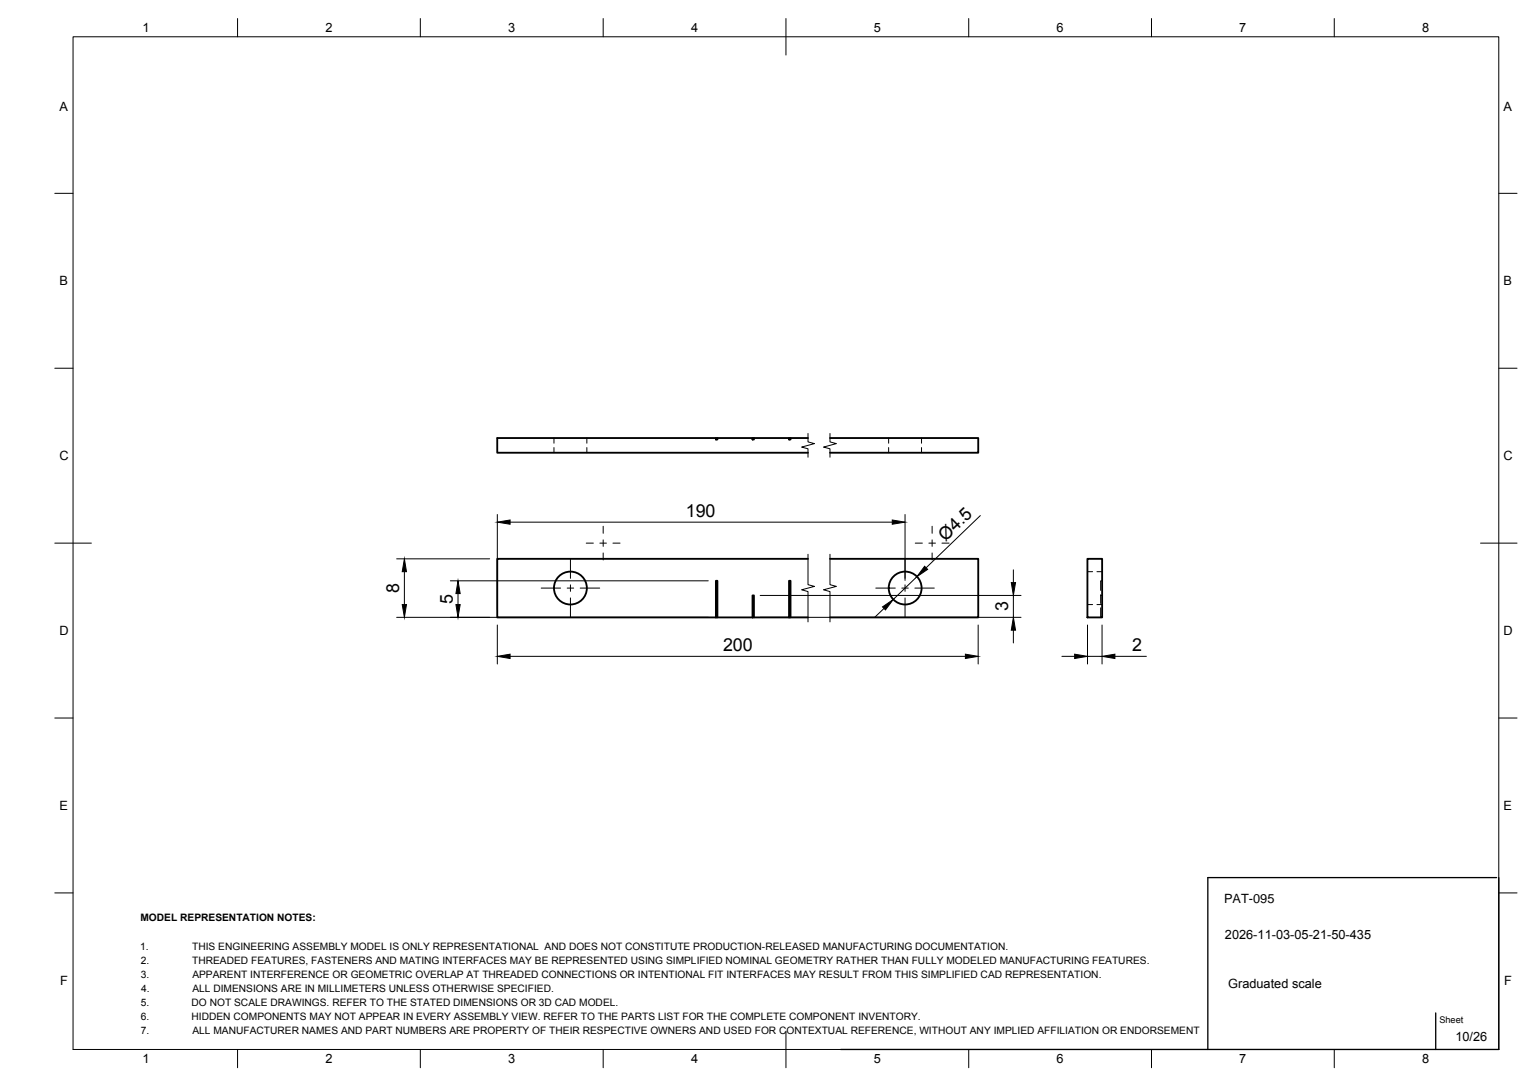
ISO-10303-21;
HEADER;
/* Generated by software containing ST-Developer
 * from STEP Tools, Inc. (www.steptools.com) 
 */

FILE_DESCRIPTION(
/* description */ ('Single-Axis Profile-Rail Linear Slide'),
/* implementation_level */ '2;1');

FILE_NAME(
/* name */ 'Graduated scale.step',
/* time_stamp */ '2026-10-27T10:47:43-07:00',
/* author */ (''),
/* organization */ (''),
/* preprocessor_version */ 'ST-DEVELOPER v20.2',
/* originating_system */ 'Autodesk Translation Framework v15.17.0.0',
/* authorisation */ '');

FILE_SCHEMA (('AUTOMOTIVE_DESIGN { 1 0 10303 214 3 1 1 }'));
ENDSEC;

DATA;
#10=MECHANICAL_DESIGN_GEOMETRIC_PRESENTATION_REPRESENTATION('',(#334),#14478);
#280=SHAPE_REPRESENTATION_RELATIONSHIP('SRR','None',#14610,#307);
#307=ADVANCED_BREP_SHAPE_REPRESENTATION('',(#361),#14454);
#334=STYLED_ITEM('',(#14845),#361);
#361=MANIFOLD_SOLID_BREP('Body1',#8594);
#418=FACE_BOUND('',#1508,.T.);
#419=FACE_BOUND('',#1509,.T.);
#420=FACE_BOUND('',#1517,.T.);
#421=FACE_BOUND('',#1518,.T.);
#502=PLANE('',#9027);
#503=PLANE('',#9028);
#504=PLANE('',#9029);
#505=PLANE('',#9030);
#506=PLANE('',#9031);
#507=PLANE('',#9032);
#508=PLANE('',#9033);
#509=PLANE('',#9034);
#510=PLANE('',#9035);
#511=PLANE('',#9036);
#512=PLANE('',#9037);
#513=PLANE('',#9038);
#514=PLANE('',#9039);
#515=PLANE('',#9040);
#516=PLANE('',#9041);
#517=PLANE('',#9042);
#518=PLANE('',#9043);
#519=PLANE('',#9044);
#520=PLANE('',#9045);
#521=PLANE('',#9046);
#522=PLANE('',#9047);
#523=PLANE('',#9048);
#524=PLANE('',#9049);
#525=PLANE('',#9050);
#526=PLANE('',#9051);
#527=PLANE('',#9052);
#528=PLANE('',#9053);
#529=PLANE('',#9054);
#530=PLANE('',#9055);
#531=PLANE('',#9056);
#532=PLANE('',#9057);
#533=PLANE('',#9058);
#534=PLANE('',#9059);
#535=PLANE('',#9060);
#536=PLANE('',#9061);
#537=PLANE('',#9062);
#538=PLANE('',#9063);
#539=PLANE('',#9064);
#540=PLANE('',#9065);
#541=PLANE('',#9066);
#542=PLANE('',#9067);
#543=PLANE('',#9068);
#544=PLANE('',#9069);
#545=PLANE('',#9070);
#546=PLANE('',#9071);
#547=PLANE('',#9072);
#548=PLANE('',#9073);
#549=PLANE('',#9074);
#550=PLANE('',#9075);
#551=PLANE('',#9076);
#552=PLANE('',#9077);
#553=PLANE('',#9078);
#554=PLANE('',#9079);
#555=PLANE('',#9080);
#556=PLANE('',#9081);
#557=PLANE('',#9082);
#558=PLANE('',#9083);
#559=PLANE('',#9084);
#560=PLANE('',#9085);
#561=PLANE('',#9086);
#562=PLANE('',#9087);
#563=PLANE('',#9088);
#564=PLANE('',#9089);
#565=PLANE('',#9090);
#566=PLANE('',#9091);
#567=PLANE('',#9092);
#568=PLANE('',#9093);
#569=PLANE('',#9094);
#570=PLANE('',#9095);
#571=PLANE('',#9096);
#572=PLANE('',#9097);
#573=PLANE('',#9098);
#574=PLANE('',#9099);
#575=PLANE('',#9100);
#576=PLANE('',#9101);
#577=PLANE('',#9102);
#578=PLANE('',#9103);
#579=PLANE('',#9104);
#580=PLANE('',#9105);
#581=PLANE('',#9106);
#582=PLANE('',#9107);
#583=PLANE('',#9108);
#584=PLANE('',#9109);
#585=PLANE('',#9110);
#586=PLANE('',#9111);
#587=PLANE('',#9112);
#588=PLANE('',#9113);
#589=PLANE('',#9114);
#590=PLANE('',#9115);
#591=PLANE('',#9116);
#592=PLANE('',#9117);
#593=PLANE('',#9118);
#594=PLANE('',#9119);
#595=PLANE('',#9120);
#596=PLANE('',#9121);
#597=PLANE('',#9122);
#598=PLANE('',#9123);
#599=PLANE('',#9124);
#600=PLANE('',#9125);
#601=PLANE('',#9126);
#602=PLANE('',#9127);
#603=PLANE('',#9128);
#604=PLANE('',#9129);
#605=PLANE('',#9130);
#606=PLANE('',#9131);
#607=PLANE('',#9132);
#608=PLANE('',#9133);
#609=PLANE('',#9134);
#610=PLANE('',#9135);
#611=PLANE('',#9136);
#612=PLANE('',#9137);
#613=PLANE('',#9138);
#614=PLANE('',#9139);
#615=PLANE('',#9140);
#616=PLANE('',#9141);
#617=PLANE('',#9142);
#618=PLANE('',#9143);
#619=PLANE('',#9150);
#620=PLANE('',#9151);
#621=PLANE('',#9152);
#622=PLANE('',#9153);
#623=PLANE('',#9154);
#896=FACE_OUTER_BOUND('',#1391,.T.);
#897=FACE_OUTER_BOUND('',#1392,.T.);
#898=FACE_OUTER_BOUND('',#1393,.T.);
#899=FACE_OUTER_BOUND('',#1394,.T.);
#900=FACE_OUTER_BOUND('',#1395,.T.);
#901=FACE_OUTER_BOUND('',#1396,.T.);
#902=FACE_OUTER_BOUND('',#1397,.T.);
#903=FACE_OUTER_BOUND('',#1398,.T.);
#904=FACE_OUTER_BOUND('',#1399,.T.);
#905=FACE_OUTER_BOUND('',#1400,.T.);
#906=FACE_OUTER_BOUND('',#1401,.T.);
#907=FACE_OUTER_BOUND('',#1402,.T.);
#908=FACE_OUTER_BOUND('',#1403,.T.);
#909=FACE_OUTER_BOUND('',#1404,.T.);
#910=FACE_OUTER_BOUND('',#1405,.T.);
#911=FACE_OUTER_BOUND('',#1406,.T.);
#912=FACE_OUTER_BOUND('',#1407,.T.);
#913=FACE_OUTER_BOUND('',#1408,.T.);
#914=FACE_OUTER_BOUND('',#1409,.T.);
#915=FACE_OUTER_BOUND('',#1410,.T.);
#916=FACE_OUTER_BOUND('',#1411,.T.);
#917=FACE_OUTER_BOUND('',#1412,.T.);
#918=FACE_OUTER_BOUND('',#1413,.T.);
#919=FACE_OUTER_BOUND('',#1414,.T.);
#920=FACE_OUTER_BOUND('',#1415,.T.);
#921=FACE_OUTER_BOUND('',#1416,.T.);
#922=FACE_OUTER_BOUND('',#1417,.T.);
#923=FACE_OUTER_BOUND('',#1418,.T.);
#924=FACE_OUTER_BOUND('',#1419,.T.);
#925=FACE_OUTER_BOUND('',#1420,.T.);
#926=FACE_OUTER_BOUND('',#1421,.T.);
#927=FACE_OUTER_BOUND('',#1422,.T.);
#928=FACE_OUTER_BOUND('',#1423,.T.);
#929=FACE_OUTER_BOUND('',#1424,.T.);
#930=FACE_OUTER_BOUND('',#1425,.T.);
#931=FACE_OUTER_BOUND('',#1426,.T.);
#932=FACE_OUTER_BOUND('',#1427,.T.);
#933=FACE_OUTER_BOUND('',#1428,.T.);
#934=FACE_OUTER_BOUND('',#1429,.T.);
#935=FACE_OUTER_BOUND('',#1430,.T.);
#936=FACE_OUTER_BOUND('',#1431,.T.);
#937=FACE_OUTER_BOUND('',#1432,.T.);
#938=FACE_OUTER_BOUND('',#1433,.T.);
#939=FACE_OUTER_BOUND('',#1434,.T.);
#940=FACE_OUTER_BOUND('',#1435,.T.);
#941=FACE_OUTER_BOUND('',#1436,.T.);
#942=FACE_OUTER_BOUND('',#1437,.T.);
#943=FACE_OUTER_BOUND('',#1438,.T.);
#944=FACE_OUTER_BOUND('',#1439,.T.);
#945=FACE_OUTER_BOUND('',#1440,.T.);
#946=FACE_OUTER_BOUND('',#1441,.T.);
#947=FACE_OUTER_BOUND('',#1442,.T.);
#948=FACE_OUTER_BOUND('',#1443,.T.);
#949=FACE_OUTER_BOUND('',#1444,.T.);
#950=FACE_OUTER_BOUND('',#1445,.T.);
#951=FACE_OUTER_BOUND('',#1446,.T.);
#952=FACE_OUTER_BOUND('',#1447,.T.);
#953=FACE_OUTER_BOUND('',#1448,.T.);
#954=FACE_OUTER_BOUND('',#1449,.T.);
#955=FACE_OUTER_BOUND('',#1450,.T.);
#956=FACE_OUTER_BOUND('',#1451,.T.);
#957=FACE_OUTER_BOUND('',#1452,.T.);
#958=FACE_OUTER_BOUND('',#1453,.T.);
#959=FACE_OUTER_BOUND('',#1454,.T.);
#960=FACE_OUTER_BOUND('',#1455,.T.);
#961=FACE_OUTER_BOUND('',#1456,.T.);
#962=FACE_OUTER_BOUND('',#1457,.T.);
#963=FACE_OUTER_BOUND('',#1458,.T.);
#964=FACE_OUTER_BOUND('',#1459,.T.);
#965=FACE_OUTER_BOUND('',#1460,.T.);
#966=FACE_OUTER_BOUND('',#1461,.T.);
#967=FACE_OUTER_BOUND('',#1462,.T.);
#968=FACE_OUTER_BOUND('',#1463,.T.);
#969=FACE_OUTER_BOUND('',#1464,.T.);
#970=FACE_OUTER_BOUND('',#1465,.T.);
#971=FACE_OUTER_BOUND('',#1466,.T.);
#972=FACE_OUTER_BOUND('',#1467,.T.);
#973=FACE_OUTER_BOUND('',#1468,.T.);
#974=FACE_OUTER_BOUND('',#1469,.T.);
#975=FACE_OUTER_BOUND('',#1470,.T.);
#976=FACE_OUTER_BOUND('',#1471,.T.);
#977=FACE_OUTER_BOUND('',#1472,.T.);
#978=FACE_OUTER_BOUND('',#1473,.T.);
#979=FACE_OUTER_BOUND('',#1474,.T.);
#980=FACE_OUTER_BOUND('',#1475,.T.);
#981=FACE_OUTER_BOUND('',#1476,.T.);
#982=FACE_OUTER_BOUND('',#1477,.T.);
#983=FACE_OUTER_BOUND('',#1478,.T.);
#984=FACE_OUTER_BOUND('',#1479,.T.);
#985=FACE_OUTER_BOUND('',#1480,.T.);
#986=FACE_OUTER_BOUND('',#1481,.T.);
#987=FACE_OUTER_BOUND('',#1482,.T.);
#988=FACE_OUTER_BOUND('',#1483,.T.);
#989=FACE_OUTER_BOUND('',#1484,.T.);
#990=FACE_OUTER_BOUND('',#1485,.T.);
#991=FACE_OUTER_BOUND('',#1486,.T.);
#992=FACE_OUTER_BOUND('',#1487,.T.);
#993=FACE_OUTER_BOUND('',#1488,.T.);
#994=FACE_OUTER_BOUND('',#1489,.T.);
#995=FACE_OUTER_BOUND('',#1490,.T.);
#996=FACE_OUTER_BOUND('',#1491,.T.);
#997=FACE_OUTER_BOUND('',#1492,.T.);
#998=FACE_OUTER_BOUND('',#1493,.T.);
#999=FACE_OUTER_BOUND('',#1494,.T.);
#1000=FACE_OUTER_BOUND('',#1495,.T.);
#1001=FACE_OUTER_BOUND('',#1496,.T.);
#1002=FACE_OUTER_BOUND('',#1497,.T.);
#1003=FACE_OUTER_BOUND('',#1498,.T.);
#1004=FACE_OUTER_BOUND('',#1499,.T.);
#1005=FACE_OUTER_BOUND('',#1500,.T.);
#1006=FACE_OUTER_BOUND('',#1501,.T.);
#1007=FACE_OUTER_BOUND('',#1502,.T.);
#1008=FACE_OUTER_BOUND('',#1503,.T.);
#1009=FACE_OUTER_BOUND('',#1504,.T.);
#1010=FACE_OUTER_BOUND('',#1505,.T.);
#1011=FACE_OUTER_BOUND('',#1506,.T.);
#1012=FACE_OUTER_BOUND('',#1507,.T.);
#1013=FACE_OUTER_BOUND('',#1510,.T.);
#1014=FACE_OUTER_BOUND('',#1511,.T.);
#1015=FACE_OUTER_BOUND('',#1512,.T.);
#1016=FACE_OUTER_BOUND('',#1513,.T.);
#1017=FACE_OUTER_BOUND('',#1514,.T.);
#1018=FACE_OUTER_BOUND('',#1515,.T.);
#1019=FACE_OUTER_BOUND('',#1516,.T.);
#1391=EDGE_LOOP('',(#6065,#6066,#6067,#6068));
#1392=EDGE_LOOP('',(#6069,#6070,#6071,#6072));
#1393=EDGE_LOOP('',(#6073,#6074,#6075,#6076));
#1394=EDGE_LOOP('',(#6077,#6078,#6079,#6080));
#1395=EDGE_LOOP('',(#6081,#6082,#6083,#6084));
#1396=EDGE_LOOP('',(#6085,#6086,#6087,#6088));
#1397=EDGE_LOOP('',(#6089,#6090,#6091,#6092));
#1398=EDGE_LOOP('',(#6093,#6094,#6095,#6096));
#1399=EDGE_LOOP('',(#6097,#6098,#6099,#6100));
#1400=EDGE_LOOP('',(#6101,#6102,#6103,#6104));
#1401=EDGE_LOOP('',(#6105,#6106,#6107,#6108));
#1402=EDGE_LOOP('',(#6109,#6110,#6111,#6112));
#1403=EDGE_LOOP('',(#6113,#6114,#6115,#6116));
#1404=EDGE_LOOP('',(#6117,#6118,#6119,#6120));
#1405=EDGE_LOOP('',(#6121,#6122,#6123,#6124));
#1406=EDGE_LOOP('',(#6125,#6126,#6127,#6128));
#1407=EDGE_LOOP('',(#6129,#6130,#6131,#6132));
#1408=EDGE_LOOP('',(#6133,#6134,#6135,#6136));
#1409=EDGE_LOOP('',(#6137,#6138,#6139,#6140));
#1410=EDGE_LOOP('',(#6141,#6142,#6143,#6144));
#1411=EDGE_LOOP('',(#6145,#6146,#6147,#6148));
#1412=EDGE_LOOP('',(#6149,#6150,#6151,#6152));
#1413=EDGE_LOOP('',(#6153,#6154,#6155,#6156));
#1414=EDGE_LOOP('',(#6157,#6158,#6159,#6160));
#1415=EDGE_LOOP('',(#6161,#6162,#6163,#6164));
#1416=EDGE_LOOP('',(#6165,#6166,#6167,#6168));
#1417=EDGE_LOOP('',(#6169,#6170,#6171,#6172));
#1418=EDGE_LOOP('',(#6173,#6174,#6175,#6176));
#1419=EDGE_LOOP('',(#6177,#6178,#6179,#6180));
#1420=EDGE_LOOP('',(#6181,#6182,#6183,#6184));
#1421=EDGE_LOOP('',(#6185,#6186,#6187,#6188));
#1422=EDGE_LOOP('',(#6189,#6190,#6191,#6192));
#1423=EDGE_LOOP('',(#6193,#6194,#6195,#6196));
#1424=EDGE_LOOP('',(#6197,#6198,#6199,#6200));
#1425=EDGE_LOOP('',(#6201,#6202,#6203,#6204));
#1426=EDGE_LOOP('',(#6205,#6206,#6207,#6208));
#1427=EDGE_LOOP('',(#6209,#6210,#6211,#6212));
#1428=EDGE_LOOP('',(#6213,#6214,#6215,#6216));
#1429=EDGE_LOOP('',(#6217,#6218,#6219,#6220));
#1430=EDGE_LOOP('',(#6221,#6222,#6223,#6224));
#1431=EDGE_LOOP('',(#6225,#6226,#6227,#6228));
#1432=EDGE_LOOP('',(#6229,#6230,#6231,#6232));
#1433=EDGE_LOOP('',(#6233,#6234,#6235,#6236));
#1434=EDGE_LOOP('',(#6237,#6238,#6239,#6240));
#1435=EDGE_LOOP('',(#6241,#6242,#6243,#6244));
#1436=EDGE_LOOP('',(#6245,#6246,#6247,#6248));
#1437=EDGE_LOOP('',(#6249,#6250,#6251,#6252));
#1438=EDGE_LOOP('',(#6253,#6254,#6255,#6256));
#1439=EDGE_LOOP('',(#6257,#6258,#6259,#6260));
#1440=EDGE_LOOP('',(#6261,#6262,#6263,#6264));
#1441=EDGE_LOOP('',(#6265,#6266,#6267,#6268));
#1442=EDGE_LOOP('',(#6269,#6270,#6271,#6272));
#1443=EDGE_LOOP('',(#6273,#6274,#6275,#6276));
#1444=EDGE_LOOP('',(#6277,#6278,#6279,#6280));
#1445=EDGE_LOOP('',(#6281,#6282,#6283,#6284));
#1446=EDGE_LOOP('',(#6285,#6286,#6287,#6288));
#1447=EDGE_LOOP('',(#6289,#6290,#6291,#6292));
#1448=EDGE_LOOP('',(#6293,#6294,#6295,#6296));
#1449=EDGE_LOOP('',(#6297,#6298,#6299,#6300));
#1450=EDGE_LOOP('',(#6301,#6302,#6303,#6304));
#1451=EDGE_LOOP('',(#6305,#6306,#6307,#6308));
#1452=EDGE_LOOP('',(#6309,#6310,#6311,#6312));
#1453=EDGE_LOOP('',(#6313,#6314,#6315,#6316));
#1454=EDGE_LOOP('',(#6317,#6318,#6319,#6320));
#1455=EDGE_LOOP('',(#6321,#6322,#6323,#6324));
#1456=EDGE_LOOP('',(#6325,#6326,#6327,#6328));
#1457=EDGE_LOOP('',(#6329,#6330,#6331,#6332));
#1458=EDGE_LOOP('',(#6333,#6334,#6335,#6336));
#1459=EDGE_LOOP('',(#6337,#6338,#6339,#6340));
#1460=EDGE_LOOP('',(#6341,#6342,#6343,#6344));
#1461=EDGE_LOOP('',(#6345,#6346,#6347,#6348));
#1462=EDGE_LOOP('',(#6349,#6350,#6351,#6352));
#1463=EDGE_LOOP('',(#6353,#6354,#6355,#6356));
#1464=EDGE_LOOP('',(#6357,#6358,#6359,#6360));
#1465=EDGE_LOOP('',(#6361,#6362,#6363,#6364));
#1466=EDGE_LOOP('',(#6365,#6366,#6367,#6368));
#1467=EDGE_LOOP('',(#6369,#6370,#6371,#6372));
#1468=EDGE_LOOP('',(#6373,#6374,#6375,#6376));
#1469=EDGE_LOOP('',(#6377,#6378,#6379,#6380));
#1470=EDGE_LOOP('',(#6381,#6382,#6383,#6384));
#1471=EDGE_LOOP('',(#6385,#6386,#6387,#6388));
#1472=EDGE_LOOP('',(#6389,#6390,#6391,#6392));
#1473=EDGE_LOOP('',(#6393,#6394,#6395,#6396));
#1474=EDGE_LOOP('',(#6397,#6398,#6399,#6400));
#1475=EDGE_LOOP('',(#6401,#6402,#6403,#6404));
#1476=EDGE_LOOP('',(#6405,#6406,#6407,#6408));
#1477=EDGE_LOOP('',(#6409,#6410,#6411,#6412));
#1478=EDGE_LOOP('',(#6413,#6414,#6415,#6416));
#1479=EDGE_LOOP('',(#6417,#6418,#6419,#6420));
#1480=EDGE_LOOP('',(#6421,#6422,#6423,#6424));
#1481=EDGE_LOOP('',(#6425,#6426,#6427,#6428));
#1482=EDGE_LOOP('',(#6429,#6430,#6431,#6432));
#1483=EDGE_LOOP('',(#6433,#6434,#6435,#6436));
#1484=EDGE_LOOP('',(#6437,#6438,#6439,#6440));
#1485=EDGE_LOOP('',(#6441,#6442,#6443,#6444));
#1486=EDGE_LOOP('',(#6445,#6446,#6447,#6448));
#1487=EDGE_LOOP('',(#6449,#6450,#6451,#6452));
#1488=EDGE_LOOP('',(#6453,#6454,#6455,#6456));
#1489=EDGE_LOOP('',(#6457,#6458,#6459,#6460));
#1490=EDGE_LOOP('',(#6461,#6462,#6463,#6464));
#1491=EDGE_LOOP('',(#6465,#6466,#6467,#6468));
#1492=EDGE_LOOP('',(#6469,#6470,#6471,#6472));
#1493=EDGE_LOOP('',(#6473,#6474,#6475,#6476));
#1494=EDGE_LOOP('',(#6477,#6478,#6479,#6480));
#1495=EDGE_LOOP('',(#6481,#6482,#6483,#6484));
#1496=EDGE_LOOP('',(#6485,#6486,#6487,#6488));
#1497=EDGE_LOOP('',(#6489,#6490,#6491,#6492));
#1498=EDGE_LOOP('',(#6493,#6494,#6495,#6496));
#1499=EDGE_LOOP('',(#6497,#6498,#6499,#6500));
#1500=EDGE_LOOP('',(#6501,#6502,#6503,#6504));
#1501=EDGE_LOOP('',(#6505,#6506,#6507,#6508));
#1502=EDGE_LOOP('',(#6509,#6510,#6511,#6512));
#1503=EDGE_LOOP('',(#6513,#6514,#6515,#6516));
#1504=EDGE_LOOP('',(#6517,#6518,#6519,#6520));
#1505=EDGE_LOOP('',(#6521,#6522,#6523,#6524));
#1506=EDGE_LOOP('',(#6525,#6526,#6527,#6528));
#1507=EDGE_LOOP('',(#6529,#6530,#6531,#6532,#6533,#6534,#6535,#6536,#6537,
#6538,#6539,#6540,#6541,#6542,#6543,#6544,#6545,#6546,#6547,#6548,#6549,
#6550,#6551,#6552,#6553,#6554,#6555,#6556,#6557,#6558,#6559,#6560,#6561,
#6562,#6563,#6564,#6565,#6566,#6567,#6568,#6569,#6570,#6571,#6572,#6573,
#6574,#6575,#6576,#6577,#6578,#6579,#6580,#6581,#6582,#6583,#6584,#6585,
#6586,#6587,#6588,#6589,#6590,#6591,#6592,#6593,#6594,#6595,#6596,#6597,
#6598,#6599,#6600,#6601,#6602,#6603,#6604,#6605,#6606,#6607,#6608,#6609,
#6610,#6611,#6612,#6613,#6614,#6615,#6616,#6617,#6618,#6619,#6620,#6621,
#6622,#6623,#6624,#6625,#6626,#6627,#6628,#6629,#6630,#6631,#6632,#6633,
#6634,#6635,#6636,#6637,#6638,#6639,#6640,#6641,#6642,#6643,#6644,#6645,
#6646,#6647,#6648));
#1508=EDGE_LOOP('',(#6649));
#1509=EDGE_LOOP('',(#6650));
#1510=EDGE_LOOP('',(#6651,#6652,#6653,#6654));
#1511=EDGE_LOOP('',(#6655,#6656,#6657,#6658));
#1512=EDGE_LOOP('',(#6659,#6660,#6661,#6662));
#1513=EDGE_LOOP('',(#6663,#6664,#6665,#6666));
#1514=EDGE_LOOP('',(#6667,#6668,#6669,#6670,#6671,#6672,#6673,#6674,#6675,
#6676,#6677,#6678,#6679,#6680,#6681,#6682,#6683,#6684,#6685,#6686,#6687,
#6688,#6689,#6690,#6691,#6692,#6693,#6694,#6695,#6696,#6697,#6698,#6699,
#6700,#6701,#6702,#6703,#6704,#6705,#6706,#6707,#6708,#6709,#6710,#6711,
#6712,#6713,#6714,#6715,#6716,#6717,#6718,#6719,#6720,#6721,#6722,#6723,
#6724,#6725,#6726,#6727,#6728,#6729,#6730,#6731,#6732,#6733,#6734,#6735,
#6736,#6737,#6738,#6739,#6740,#6741,#6742,#6743,#6744,#6745,#6746,#6747,
#6748,#6749,#6750,#6751,#6752,#6753,#6754,#6755,#6756,#6757,#6758,#6759,
#6760,#6761,#6762,#6763,#6764,#6765,#6766,#6767,#6768,#6769,#6770,#6771,
#6772,#6773,#6774,#6775,#6776,#6777,#6778,#6779,#6780,#6781,#6782,#6783,
#6784,#6785,#6786));
#1515=EDGE_LOOP('',(#6787,#6788,#6789,#6790));
#1516=EDGE_LOOP('',(#6791,#6792,#6793,#6794));
#1517=EDGE_LOOP('',(#6795));
#1518=EDGE_LOOP('',(#6796));
#1922=LINE('',#12273,#2893);
#1923=LINE('',#12275,#2894);
#1924=LINE('',#12277,#2895);
#1925=LINE('',#12278,#2896);
#1926=LINE('',#12281,#2897);
#1927=LINE('',#12283,#2898);
#1928=LINE('',#12284,#2899);
#1929=LINE('',#12287,#2900);
#1930=LINE('',#12289,#2901);
#1931=LINE('',#12290,#2902);
#1932=LINE('',#12292,#2903);
#1933=LINE('',#12296,#2904);
#1934=LINE('',#12298,#2905);
#1935=LINE('',#12300,#2906);
#1936=LINE('',#12301,#2907);
#1937=LINE('',#12304,#2908);
#1938=LINE('',#12306,#2909);
#1939=LINE('',#12307,#2910);
#1940=LINE('',#12310,#2911);
#1941=LINE('',#12312,#2912);
#1942=LINE('',#12313,#2913);
#1943=LINE('',#12315,#2914);
#1944=LINE('',#12319,#2915);
#1945=LINE('',#12321,#2916);
#1946=LINE('',#12323,#2917);
#1947=LINE('',#12324,#2918);
#1948=LINE('',#12327,#2919);
#1949=LINE('',#12329,#2920);
#1950=LINE('',#12330,#2921);
#1951=LINE('',#12333,#2922);
#1952=LINE('',#12335,#2923);
#1953=LINE('',#12336,#2924);
#1954=LINE('',#12338,#2925);
#1955=LINE('',#12342,#2926);
#1956=LINE('',#12344,#2927);
#1957=LINE('',#12346,#2928);
#1958=LINE('',#12347,#2929);
#1959=LINE('',#12350,#2930);
#1960=LINE('',#12352,#2931);
#1961=LINE('',#12353,#2932);
#1962=LINE('',#12356,#2933);
#1963=LINE('',#12358,#2934);
#1964=LINE('',#12359,#2935);
#1965=LINE('',#12361,#2936);
#1966=LINE('',#12365,#2937);
#1967=LINE('',#12367,#2938);
#1968=LINE('',#12369,#2939);
#1969=LINE('',#12370,#2940);
#1970=LINE('',#12373,#2941);
#1971=LINE('',#12375,#2942);
#1972=LINE('',#12376,#2943);
#1973=LINE('',#12379,#2944);
#1974=LINE('',#12381,#2945);
#1975=LINE('',#12382,#2946);
#1976=LINE('',#12384,#2947);
#1977=LINE('',#12388,#2948);
#1978=LINE('',#12390,#2949);
#1979=LINE('',#12392,#2950);
#1980=LINE('',#12393,#2951);
#1981=LINE('',#12396,#2952);
#1982=LINE('',#12398,#2953);
#1983=LINE('',#12399,#2954);
#1984=LINE('',#12402,#2955);
#1985=LINE('',#12404,#2956);
#1986=LINE('',#12405,#2957);
#1987=LINE('',#12407,#2958);
#1988=LINE('',#12411,#2959);
#1989=LINE('',#12413,#2960);
#1990=LINE('',#12415,#2961);
#1991=LINE('',#12416,#2962);
#1992=LINE('',#12419,#2963);
#1993=LINE('',#12421,#2964);
#1994=LINE('',#12422,#2965);
#1995=LINE('',#12425,#2966);
#1996=LINE('',#12427,#2967);
#1997=LINE('',#12428,#2968);
#1998=LINE('',#12430,#2969);
#1999=LINE('',#12434,#2970);
#2000=LINE('',#12436,#2971);
#2001=LINE('',#12438,#2972);
#2002=LINE('',#12439,#2973);
#2003=LINE('',#12442,#2974);
#2004=LINE('',#12444,#2975);
#2005=LINE('',#12445,#2976);
#2006=LINE('',#12448,#2977);
#2007=LINE('',#12450,#2978);
#2008=LINE('',#12451,#2979);
#2009=LINE('',#12453,#2980);
#2010=LINE('',#12457,#2981);
#2011=LINE('',#12459,#2982);
#2012=LINE('',#12461,#2983);
#2013=LINE('',#12462,#2984);
#2014=LINE('',#12465,#2985);
#2015=LINE('',#12467,#2986);
#2016=LINE('',#12468,#2987);
#2017=LINE('',#12471,#2988);
#2018=LINE('',#12473,#2989);
#2019=LINE('',#12474,#2990);
#2020=LINE('',#12476,#2991);
#2021=LINE('',#12480,#2992);
#2022=LINE('',#12482,#2993);
#2023=LINE('',#12484,#2994);
#2024=LINE('',#12485,#2995);
#2025=LINE('',#12488,#2996);
#2026=LINE('',#12490,#2997);
#2027=LINE('',#12491,#2998);
#2028=LINE('',#12494,#2999);
#2029=LINE('',#12496,#3000);
#2030=LINE('',#12497,#3001);
#2031=LINE('',#12499,#3002);
#2032=LINE('',#12503,#3003);
#2033=LINE('',#12505,#3004);
#2034=LINE('',#12507,#3005);
#2035=LINE('',#12508,#3006);
#2036=LINE('',#12511,#3007);
#2037=LINE('',#12513,#3008);
#2038=LINE('',#12514,#3009);
#2039=LINE('',#12517,#3010);
#2040=LINE('',#12519,#3011);
#2041=LINE('',#12520,#3012);
#2042=LINE('',#12522,#3013);
#2043=LINE('',#12526,#3014);
#2044=LINE('',#12528,#3015);
#2045=LINE('',#12530,#3016);
#2046=LINE('',#12531,#3017);
#2047=LINE('',#12534,#3018);
#2048=LINE('',#12536,#3019);
#2049=LINE('',#12537,#3020);
#2050=LINE('',#12540,#3021);
#2051=LINE('',#12542,#3022);
#2052=LINE('',#12543,#3023);
#2053=LINE('',#12545,#3024);
#2054=LINE('',#12549,#3025);
#2055=LINE('',#12551,#3026);
#2056=LINE('',#12553,#3027);
#2057=LINE('',#12554,#3028);
#2058=LINE('',#12557,#3029);
#2059=LINE('',#12559,#3030);
#2060=LINE('',#12560,#3031);
#2061=LINE('',#12563,#3032);
#2062=LINE('',#12565,#3033);
#2063=LINE('',#12566,#3034);
#2064=LINE('',#12568,#3035);
#2065=LINE('',#12572,#3036);
#2066=LINE('',#12574,#3037);
#2067=LINE('',#12576,#3038);
#2068=LINE('',#12577,#3039);
#2069=LINE('',#12580,#3040);
#2070=LINE('',#12582,#3041);
#2071=LINE('',#12583,#3042);
#2072=LINE('',#12586,#3043);
#2073=LINE('',#12588,#3044);
#2074=LINE('',#12589,#3045);
#2075=LINE('',#12591,#3046);
#2076=LINE('',#12595,#3047);
#2077=LINE('',#12597,#3048);
#2078=LINE('',#12599,#3049);
#2079=LINE('',#12600,#3050);
#2080=LINE('',#12603,#3051);
#2081=LINE('',#12605,#3052);
#2082=LINE('',#12606,#3053);
#2083=LINE('',#12609,#3054);
#2084=LINE('',#12611,#3055);
#2085=LINE('',#12612,#3056);
#2086=LINE('',#12614,#3057);
#2087=LINE('',#12618,#3058);
#2088=LINE('',#12620,#3059);
#2089=LINE('',#12622,#3060);
#2090=LINE('',#12623,#3061);
#2091=LINE('',#12626,#3062);
#2092=LINE('',#12628,#3063);
#2093=LINE('',#12629,#3064);
#2094=LINE('',#12632,#3065);
#2095=LINE('',#12634,#3066);
#2096=LINE('',#12635,#3067);
#2097=LINE('',#12637,#3068);
#2098=LINE('',#12641,#3069);
#2099=LINE('',#12643,#3070);
#2100=LINE('',#12645,#3071);
#2101=LINE('',#12646,#3072);
#2102=LINE('',#12649,#3073);
#2103=LINE('',#12651,#3074);
#2104=LINE('',#12652,#3075);
#2105=LINE('',#12655,#3076);
#2106=LINE('',#12657,#3077);
#2107=LINE('',#12658,#3078);
#2108=LINE('',#12660,#3079);
#2109=LINE('',#12664,#3080);
#2110=LINE('',#12666,#3081);
#2111=LINE('',#12668,#3082);
#2112=LINE('',#12669,#3083);
#2113=LINE('',#12672,#3084);
#2114=LINE('',#12674,#3085);
#2115=LINE('',#12675,#3086);
#2116=LINE('',#12678,#3087);
#2117=LINE('',#12680,#3088);
#2118=LINE('',#12681,#3089);
#2119=LINE('',#12683,#3090);
#2120=LINE('',#12687,#3091);
#2121=LINE('',#12689,#3092);
#2122=LINE('',#12691,#3093);
#2123=LINE('',#12692,#3094);
#2124=LINE('',#12695,#3095);
#2125=LINE('',#12697,#3096);
#2126=LINE('',#12698,#3097);
#2127=LINE('',#12701,#3098);
#2128=LINE('',#12703,#3099);
#2129=LINE('',#12704,#3100);
#2130=LINE('',#12706,#3101);
#2131=LINE('',#12710,#3102);
#2132=LINE('',#12712,#3103);
#2133=LINE('',#12714,#3104);
#2134=LINE('',#12715,#3105);
#2135=LINE('',#12718,#3106);
#2136=LINE('',#12720,#3107);
#2137=LINE('',#12721,#3108);
#2138=LINE('',#12724,#3109);
#2139=LINE('',#12726,#3110);
#2140=LINE('',#12727,#3111);
#2141=LINE('',#12729,#3112);
#2142=LINE('',#12733,#3113);
#2143=LINE('',#12735,#3114);
#2144=LINE('',#12737,#3115);
#2145=LINE('',#12738,#3116);
#2146=LINE('',#12741,#3117);
#2147=LINE('',#12743,#3118);
#2148=LINE('',#12744,#3119);
#2149=LINE('',#12747,#3120);
#2150=LINE('',#12749,#3121);
#2151=LINE('',#12750,#3122);
#2152=LINE('',#12752,#3123);
#2153=LINE('',#12756,#3124);
#2154=LINE('',#12758,#3125);
#2155=LINE('',#12760,#3126);
#2156=LINE('',#12761,#3127);
#2157=LINE('',#12764,#3128);
#2158=LINE('',#12766,#3129);
#2159=LINE('',#12767,#3130);
#2160=LINE('',#12770,#3131);
#2161=LINE('',#12772,#3132);
#2162=LINE('',#12773,#3133);
#2163=LINE('',#12775,#3134);
#2164=LINE('',#12779,#3135);
#2165=LINE('',#12781,#3136);
#2166=LINE('',#12783,#3137);
#2167=LINE('',#12784,#3138);
#2168=LINE('',#12787,#3139);
#2169=LINE('',#12789,#3140);
#2170=LINE('',#12790,#3141);
#2171=LINE('',#12793,#3142);
#2172=LINE('',#12795,#3143);
#2173=LINE('',#12796,#3144);
#2174=LINE('',#12798,#3145);
#2175=LINE('',#12802,#3146);
#2176=LINE('',#12804,#3147);
#2177=LINE('',#12806,#3148);
#2178=LINE('',#12807,#3149);
#2179=LINE('',#12810,#3150);
#2180=LINE('',#12812,#3151);
#2181=LINE('',#12813,#3152);
#2182=LINE('',#12816,#3153);
#2183=LINE('',#12818,#3154);
#2184=LINE('',#12819,#3155);
#2185=LINE('',#12821,#3156);
#2186=LINE('',#12825,#3157);
#2187=LINE('',#12827,#3158);
#2188=LINE('',#12829,#3159);
#2189=LINE('',#12830,#3160);
#2190=LINE('',#12833,#3161);
#2191=LINE('',#12835,#3162);
#2192=LINE('',#12836,#3163);
#2193=LINE('',#12839,#3164);
#2194=LINE('',#12841,#3165);
#2195=LINE('',#12842,#3166);
#2196=LINE('',#12844,#3167);
#2197=LINE('',#12848,#3168);
#2198=LINE('',#12850,#3169);
#2199=LINE('',#12852,#3170);
#2200=LINE('',#12853,#3171);
#2201=LINE('',#12856,#3172);
#2202=LINE('',#12858,#3173);
#2203=LINE('',#12859,#3174);
#2204=LINE('',#12862,#3175);
#2205=LINE('',#12864,#3176);
#2206=LINE('',#12865,#3177);
#2207=LINE('',#12867,#3178);
#2208=LINE('',#12871,#3179);
#2209=LINE('',#12873,#3180);
#2210=LINE('',#12875,#3181);
#2211=LINE('',#12876,#3182);
#2212=LINE('',#12879,#3183);
#2213=LINE('',#12881,#3184);
#2214=LINE('',#12882,#3185);
#2215=LINE('',#12885,#3186);
#2216=LINE('',#12887,#3187);
#2217=LINE('',#12888,#3188);
#2218=LINE('',#12890,#3189);
#2219=LINE('',#12894,#3190);
#2220=LINE('',#12896,#3191);
#2221=LINE('',#12898,#3192);
#2222=LINE('',#12899,#3193);
#2223=LINE('',#12902,#3194);
#2224=LINE('',#12904,#3195);
#2225=LINE('',#12905,#3196);
#2226=LINE('',#12908,#3197);
#2227=LINE('',#12910,#3198);
#2228=LINE('',#12911,#3199);
#2229=LINE('',#12913,#3200);
#2230=LINE('',#12917,#3201);
#2231=LINE('',#12919,#3202);
#2232=LINE('',#12921,#3203);
#2233=LINE('',#12922,#3204);
#2234=LINE('',#12925,#3205);
#2235=LINE('',#12927,#3206);
#2236=LINE('',#12928,#3207);
#2237=LINE('',#12931,#3208);
#2238=LINE('',#12933,#3209);
#2239=LINE('',#12934,#3210);
#2240=LINE('',#12936,#3211);
#2241=LINE('',#12938,#3212);
#2242=LINE('',#12940,#3213);
#2243=LINE('',#12942,#3214);
#2244=LINE('',#12944,#3215);
#2245=LINE('',#12946,#3216);
#2246=LINE('',#12947,#3217);
#2247=LINE('',#12948,#3218);
#2248=LINE('',#12949,#3219);
#2249=LINE('',#12950,#3220);
#2250=LINE('',#12951,#3221);
#2251=LINE('',#12952,#3222);
#2252=LINE('',#12953,#3223);
#2253=LINE('',#12954,#3224);
#2254=LINE('',#12955,#3225);
#2255=LINE('',#12956,#3226);
#2256=LINE('',#12957,#3227);
#2257=LINE('',#12958,#3228);
#2258=LINE('',#12959,#3229);
#2259=LINE('',#12960,#3230);
#2260=LINE('',#12961,#3231);
#2261=LINE('',#12962,#3232);
#2262=LINE('',#12963,#3233);
#2263=LINE('',#12964,#3234);
#2264=LINE('',#12965,#3235);
#2265=LINE('',#12966,#3236);
#2266=LINE('',#12967,#3237);
#2267=LINE('',#12968,#3238);
#2268=LINE('',#12969,#3239);
#2269=LINE('',#12970,#3240);
#2270=LINE('',#12971,#3241);
#2271=LINE('',#12972,#3242);
#2272=LINE('',#12973,#3243);
#2273=LINE('',#12974,#3244);
#2274=LINE('',#12982,#3245);
#2275=LINE('',#12986,#3246);
#2276=LINE('',#12990,#3247);
#2277=LINE('',#12991,#3248);
#2278=LINE('',#12992,#3249);
#2279=LINE('',#12995,#3250);
#2280=LINE('',#12996,#3251);
#2281=LINE('',#12999,#3252);
#2282=LINE('',#13000,#3253);
#2283=LINE('',#13002,#3254);
#2893=VECTOR('',#9921,1.);
#2894=VECTOR('',#9922,1.);
#2895=VECTOR('',#9923,1.);
#2896=VECTOR('',#9924,1.);
#2897=VECTOR('',#9927,1.);
#2898=VECTOR('',#9928,1.);
#2899=VECTOR('',#9929,1.);
#2900=VECTOR('',#9932,1.);
#2901=VECTOR('',#9933,1.);
#2902=VECTOR('',#9934,1.);
#2903=VECTOR('',#9937,1.);
#2904=VECTOR('',#9940,1.);
#2905=VECTOR('',#9941,1.);
#2906=VECTOR('',#9942,1.);
#2907=VECTOR('',#9943,1.);
#2908=VECTOR('',#9946,1.);
#2909=VECTOR('',#9947,1.);
#2910=VECTOR('',#9948,1.);
#2911=VECTOR('',#9951,1.);
#2912=VECTOR('',#9952,1.);
#2913=VECTOR('',#9953,1.);
#2914=VECTOR('',#9956,1.);
#2915=VECTOR('',#9959,1.);
#2916=VECTOR('',#9960,1.);
#2917=VECTOR('',#9961,1.);
#2918=VECTOR('',#9962,1.);
#2919=VECTOR('',#9965,1.);
#2920=VECTOR('',#9966,1.);
#2921=VECTOR('',#9967,1.);
#2922=VECTOR('',#9970,1.);
#2923=VECTOR('',#9971,1.);
#2924=VECTOR('',#9972,1.);
#2925=VECTOR('',#9975,1.);
#2926=VECTOR('',#9978,1.);
#2927=VECTOR('',#9979,1.);
#2928=VECTOR('',#9980,1.);
#2929=VECTOR('',#9981,1.);
#2930=VECTOR('',#9984,1.);
#2931=VECTOR('',#9985,1.);
#2932=VECTOR('',#9986,1.);
#2933=VECTOR('',#9989,1.);
#2934=VECTOR('',#9990,1.);
#2935=VECTOR('',#9991,1.);
#2936=VECTOR('',#9994,1.);
#2937=VECTOR('',#9997,1.);
#2938=VECTOR('',#9998,1.);
#2939=VECTOR('',#9999,1.);
#2940=VECTOR('',#10000,1.);
#2941=VECTOR('',#10003,1.);
#2942=VECTOR('',#10004,1.);
#2943=VECTOR('',#10005,1.);
#2944=VECTOR('',#10008,1.);
#2945=VECTOR('',#10009,1.);
#2946=VECTOR('',#10010,1.);
#2947=VECTOR('',#10013,1.);
#2948=VECTOR('',#10016,1.);
#2949=VECTOR('',#10017,1.);
#2950=VECTOR('',#10018,1.);
#2951=VECTOR('',#10019,1.);
#2952=VECTOR('',#10022,1.);
#2953=VECTOR('',#10023,1.);
#2954=VECTOR('',#10024,1.);
#2955=VECTOR('',#10027,1.);
#2956=VECTOR('',#10028,1.);
#2957=VECTOR('',#10029,1.);
#2958=VECTOR('',#10032,1.);
#2959=VECTOR('',#10035,1.);
#2960=VECTOR('',#10036,1.);
#2961=VECTOR('',#10037,1.);
#2962=VECTOR('',#10038,1.);
#2963=VECTOR('',#10041,1.);
#2964=VECTOR('',#10042,1.);
#2965=VECTOR('',#10043,1.);
#2966=VECTOR('',#10046,1.);
#2967=VECTOR('',#10047,1.);
#2968=VECTOR('',#10048,1.);
#2969=VECTOR('',#10051,1.);
#2970=VECTOR('',#10054,1.);
#2971=VECTOR('',#10055,1.);
#2972=VECTOR('',#10056,1.);
#2973=VECTOR('',#10057,1.);
#2974=VECTOR('',#10060,1.);
#2975=VECTOR('',#10061,1.);
#2976=VECTOR('',#10062,1.);
#2977=VECTOR('',#10065,1.);
#2978=VECTOR('',#10066,1.);
#2979=VECTOR('',#10067,1.);
#2980=VECTOR('',#10070,1.);
#2981=VECTOR('',#10073,1.);
#2982=VECTOR('',#10074,1.);
#2983=VECTOR('',#10075,1.);
#2984=VECTOR('',#10076,1.);
#2985=VECTOR('',#10079,1.);
#2986=VECTOR('',#10080,1.);
#2987=VECTOR('',#10081,1.);
#2988=VECTOR('',#10084,1.);
#2989=VECTOR('',#10085,1.);
#2990=VECTOR('',#10086,1.);
#2991=VECTOR('',#10089,1.);
#2992=VECTOR('',#10092,1.);
#2993=VECTOR('',#10093,1.);
#2994=VECTOR('',#10094,1.);
#2995=VECTOR('',#10095,1.);
#2996=VECTOR('',#10098,1.);
#2997=VECTOR('',#10099,1.);
#2998=VECTOR('',#10100,1.);
#2999=VECTOR('',#10103,1.);
#3000=VECTOR('',#10104,1.);
#3001=VECTOR('',#10105,1.);
#3002=VECTOR('',#10108,1.);
#3003=VECTOR('',#10111,1.);
#3004=VECTOR('',#10112,1.);
#3005=VECTOR('',#10113,1.);
#3006=VECTOR('',#10114,1.);
#3007=VECTOR('',#10117,1.);
#3008=VECTOR('',#10118,1.);
#3009=VECTOR('',#10119,1.);
#3010=VECTOR('',#10122,1.);
#3011=VECTOR('',#10123,1.);
#3012=VECTOR('',#10124,1.);
#3013=VECTOR('',#10127,1.);
#3014=VECTOR('',#10130,1.);
#3015=VECTOR('',#10131,1.);
#3016=VECTOR('',#10132,1.);
#3017=VECTOR('',#10133,1.);
#3018=VECTOR('',#10136,1.);
#3019=VECTOR('',#10137,1.);
#3020=VECTOR('',#10138,1.);
#3021=VECTOR('',#10141,1.);
#3022=VECTOR('',#10142,1.);
#3023=VECTOR('',#10143,1.);
#3024=VECTOR('',#10146,1.);
#3025=VECTOR('',#10149,1.);
#3026=VECTOR('',#10150,1.);
#3027=VECTOR('',#10151,1.);
#3028=VECTOR('',#10152,1.);
#3029=VECTOR('',#10155,1.);
#3030=VECTOR('',#10156,1.);
#3031=VECTOR('',#10157,1.);
#3032=VECTOR('',#10160,1.);
#3033=VECTOR('',#10161,1.);
#3034=VECTOR('',#10162,1.);
#3035=VECTOR('',#10165,1.);
#3036=VECTOR('',#10168,1.);
#3037=VECTOR('',#10169,1.);
#3038=VECTOR('',#10170,1.);
#3039=VECTOR('',#10171,1.);
#3040=VECTOR('',#10174,1.);
#3041=VECTOR('',#10175,1.);
#3042=VECTOR('',#10176,1.);
#3043=VECTOR('',#10179,1.);
#3044=VECTOR('',#10180,1.);
#3045=VECTOR('',#10181,1.);
#3046=VECTOR('',#10184,1.);
#3047=VECTOR('',#10187,1.);
#3048=VECTOR('',#10188,1.);
#3049=VECTOR('',#10189,1.);
#3050=VECTOR('',#10190,1.);
#3051=VECTOR('',#10193,1.);
#3052=VECTOR('',#10194,1.);
#3053=VECTOR('',#10195,1.);
#3054=VECTOR('',#10198,1.);
#3055=VECTOR('',#10199,1.);
#3056=VECTOR('',#10200,1.);
#3057=VECTOR('',#10203,1.);
#3058=VECTOR('',#10206,1.);
#3059=VECTOR('',#10207,1.);
#3060=VECTOR('',#10208,1.);
#3061=VECTOR('',#10209,1.);
#3062=VECTOR('',#10212,1.);
#3063=VECTOR('',#10213,1.);
#3064=VECTOR('',#10214,1.);
#3065=VECTOR('',#10217,1.);
#3066=VECTOR('',#10218,1.);
#3067=VECTOR('',#10219,1.);
#3068=VECTOR('',#10222,1.);
#3069=VECTOR('',#10225,1.);
#3070=VECTOR('',#10226,1.);
#3071=VECTOR('',#10227,1.);
#3072=VECTOR('',#10228,1.);
#3073=VECTOR('',#10231,1.);
#3074=VECTOR('',#10232,1.);
#3075=VECTOR('',#10233,1.);
#3076=VECTOR('',#10236,1.);
#3077=VECTOR('',#10237,1.);
#3078=VECTOR('',#10238,1.);
#3079=VECTOR('',#10241,1.);
#3080=VECTOR('',#10244,1.);
#3081=VECTOR('',#10245,1.);
#3082=VECTOR('',#10246,1.);
#3083=VECTOR('',#10247,1.);
#3084=VECTOR('',#10250,1.);
#3085=VECTOR('',#10251,1.);
#3086=VECTOR('',#10252,1.);
#3087=VECTOR('',#10255,1.);
#3088=VECTOR('',#10256,1.);
#3089=VECTOR('',#10257,1.);
#3090=VECTOR('',#10260,1.);
#3091=VECTOR('',#10263,1.);
#3092=VECTOR('',#10264,1.);
#3093=VECTOR('',#10265,1.);
#3094=VECTOR('',#10266,1.);
#3095=VECTOR('',#10269,1.);
#3096=VECTOR('',#10270,1.);
#3097=VECTOR('',#10271,1.);
#3098=VECTOR('',#10274,1.);
#3099=VECTOR('',#10275,1.);
#3100=VECTOR('',#10276,1.);
#3101=VECTOR('',#10279,1.);
#3102=VECTOR('',#10282,1.);
#3103=VECTOR('',#10283,1.);
#3104=VECTOR('',#10284,1.);
#3105=VECTOR('',#10285,1.);
#3106=VECTOR('',#10288,1.);
#3107=VECTOR('',#10289,1.);
#3108=VECTOR('',#10290,1.);
#3109=VECTOR('',#10293,1.);
#3110=VECTOR('',#10294,1.);
#3111=VECTOR('',#10295,1.);
#3112=VECTOR('',#10298,1.);
#3113=VECTOR('',#10301,1.);
#3114=VECTOR('',#10302,1.);
#3115=VECTOR('',#10303,1.);
#3116=VECTOR('',#10304,1.);
#3117=VECTOR('',#10307,1.);
#3118=VECTOR('',#10308,1.);
#3119=VECTOR('',#10309,1.);
#3120=VECTOR('',#10312,1.);
#3121=VECTOR('',#10313,1.);
#3122=VECTOR('',#10314,1.);
#3123=VECTOR('',#10317,1.);
#3124=VECTOR('',#10320,1.);
#3125=VECTOR('',#10321,1.);
#3126=VECTOR('',#10322,1.);
#3127=VECTOR('',#10323,1.);
#3128=VECTOR('',#10326,1.);
#3129=VECTOR('',#10327,1.);
#3130=VECTOR('',#10328,1.);
#3131=VECTOR('',#10331,1.);
#3132=VECTOR('',#10332,1.);
#3133=VECTOR('',#10333,1.);
#3134=VECTOR('',#10336,1.);
#3135=VECTOR('',#10339,1.);
#3136=VECTOR('',#10340,1.);
#3137=VECTOR('',#10341,1.);
#3138=VECTOR('',#10342,1.);
#3139=VECTOR('',#10345,1.);
#3140=VECTOR('',#10346,1.);
#3141=VECTOR('',#10347,1.);
#3142=VECTOR('',#10350,1.);
#3143=VECTOR('',#10351,1.);
#3144=VECTOR('',#10352,1.);
#3145=VECTOR('',#10355,1.);
#3146=VECTOR('',#10358,1.);
#3147=VECTOR('',#10359,1.);
#3148=VECTOR('',#10360,1.);
#3149=VECTOR('',#10361,1.);
#3150=VECTOR('',#10364,1.);
#3151=VECTOR('',#10365,1.);
#3152=VECTOR('',#10366,1.);
#3153=VECTOR('',#10369,1.);
#3154=VECTOR('',#10370,1.);
#3155=VECTOR('',#10371,1.);
#3156=VECTOR('',#10374,1.);
#3157=VECTOR('',#10377,1.);
#3158=VECTOR('',#10378,1.);
#3159=VECTOR('',#10379,1.);
#3160=VECTOR('',#10380,1.);
#3161=VECTOR('',#10383,1.);
#3162=VECTOR('',#10384,1.);
#3163=VECTOR('',#10385,1.);
#3164=VECTOR('',#10388,1.);
#3165=VECTOR('',#10389,1.);
#3166=VECTOR('',#10390,1.);
#3167=VECTOR('',#10393,1.);
#3168=VECTOR('',#10396,1.);
#3169=VECTOR('',#10397,1.);
#3170=VECTOR('',#10398,1.);
#3171=VECTOR('',#10399,1.);
#3172=VECTOR('',#10402,1.);
#3173=VECTOR('',#10403,1.);
#3174=VECTOR('',#10404,1.);
#3175=VECTOR('',#10407,1.);
#3176=VECTOR('',#10408,1.);
#3177=VECTOR('',#10409,1.);
#3178=VECTOR('',#10412,1.);
#3179=VECTOR('',#10415,1.);
#3180=VECTOR('',#10416,1.);
#3181=VECTOR('',#10417,1.);
#3182=VECTOR('',#10418,1.);
#3183=VECTOR('',#10421,1.);
#3184=VECTOR('',#10422,1.);
#3185=VECTOR('',#10423,1.);
#3186=VECTOR('',#10426,1.);
#3187=VECTOR('',#10427,1.);
#3188=VECTOR('',#10428,1.);
#3189=VECTOR('',#10431,1.);
#3190=VECTOR('',#10434,1.);
#3191=VECTOR('',#10435,1.);
#3192=VECTOR('',#10436,1.);
#3193=VECTOR('',#10437,1.);
#3194=VECTOR('',#10440,1.);
#3195=VECTOR('',#10441,1.);
#3196=VECTOR('',#10442,1.);
#3197=VECTOR('',#10445,1.);
#3198=VECTOR('',#10446,1.);
#3199=VECTOR('',#10447,1.);
#3200=VECTOR('',#10450,1.);
#3201=VECTOR('',#10453,1.);
#3202=VECTOR('',#10454,1.);
#3203=VECTOR('',#10455,1.);
#3204=VECTOR('',#10456,1.);
#3205=VECTOR('',#10459,1.);
#3206=VECTOR('',#10460,1.);
#3207=VECTOR('',#10461,1.);
#3208=VECTOR('',#10464,1.);
#3209=VECTOR('',#10465,1.);
#3210=VECTOR('',#10466,1.);
#3211=VECTOR('',#10469,1.);
#3212=VECTOR('',#10472,1.);
#3213=VECTOR('',#10473,1.);
#3214=VECTOR('',#10474,1.);
#3215=VECTOR('',#10475,1.);
#3216=VECTOR('',#10476,1.);
#3217=VECTOR('',#10477,1.);
#3218=VECTOR('',#10478,1.);
#3219=VECTOR('',#10479,1.);
#3220=VECTOR('',#10480,1.);
#3221=VECTOR('',#10481,1.);
#3222=VECTOR('',#10482,1.);
#3223=VECTOR('',#10483,1.);
#3224=VECTOR('',#10484,1.);
#3225=VECTOR('',#10485,1.);
#3226=VECTOR('',#10486,1.);
#3227=VECTOR('',#10487,1.);
#3228=VECTOR('',#10488,1.);
#3229=VECTOR('',#10489,1.);
#3230=VECTOR('',#10490,1.);
#3231=VECTOR('',#10491,1.);
#3232=VECTOR('',#10492,1.);
#3233=VECTOR('',#10493,1.);
#3234=VECTOR('',#10494,1.);
#3235=VECTOR('',#10495,1.);
#3236=VECTOR('',#10496,1.);
#3237=VECTOR('',#10497,1.);
#3238=VECTOR('',#10498,1.);
#3239=VECTOR('',#10499,1.);
#3240=VECTOR('',#10500,1.);
#3241=VECTOR('',#10501,1.);
#3242=VECTOR('',#10502,1.);
#3243=VECTOR('',#10503,1.);
#3244=VECTOR('',#10504,1.);
#3245=VECTOR('',#10513,0.225);
#3246=VECTOR('',#10518,0.225000000000001);
#3247=VECTOR('',#10521,1.);
#3248=VECTOR('',#10522,1.);
#3249=VECTOR('',#10523,1.);
#3250=VECTOR('',#10526,1.);
#3251=VECTOR('',#10527,1.);
#3252=VECTOR('',#10530,1.);
#3253=VECTOR('',#10531,1.);
#3254=VECTOR('',#10534,1.);
#3826=CIRCLE('',#9144,0.225000000000001);
#3827=CIRCLE('',#9145,0.225);
#3828=CIRCLE('',#9147,0.225);
#3829=CIRCLE('',#9149,0.225000000000001);
#4022=VERTEX_POINT('',#12271);
#4023=VERTEX_POINT('',#12272);
#4024=VERTEX_POINT('',#12274);
#4025=VERTEX_POINT('',#12276);
#4026=VERTEX_POINT('',#12280);
#4027=VERTEX_POINT('',#12282);
#4028=VERTEX_POINT('',#12286);
#4029=VERTEX_POINT('',#12288);
#4030=VERTEX_POINT('',#12294);
#4031=VERTEX_POINT('',#12295);
#4032=VERTEX_POINT('',#12297);
#4033=VERTEX_POINT('',#12299);
#4034=VERTEX_POINT('',#12303);
#4035=VERTEX_POINT('',#12305);
#4036=VERTEX_POINT('',#12309);
#4037=VERTEX_POINT('',#12311);
#4038=VERTEX_POINT('',#12317);
#4039=VERTEX_POINT('',#12318);
#4040=VERTEX_POINT('',#12320);
#4041=VERTEX_POINT('',#12322);
#4042=VERTEX_POINT('',#12326);
#4043=VERTEX_POINT('',#12328);
#4044=VERTEX_POINT('',#12332);
#4045=VERTEX_POINT('',#12334);
#4046=VERTEX_POINT('',#12340);
#4047=VERTEX_POINT('',#12341);
#4048=VERTEX_POINT('',#12343);
#4049=VERTEX_POINT('',#12345);
#4050=VERTEX_POINT('',#12349);
#4051=VERTEX_POINT('',#12351);
#4052=VERTEX_POINT('',#12355);
#4053=VERTEX_POINT('',#12357);
#4054=VERTEX_POINT('',#12363);
#4055=VERTEX_POINT('',#12364);
#4056=VERTEX_POINT('',#12366);
#4057=VERTEX_POINT('',#12368);
#4058=VERTEX_POINT('',#12372);
#4059=VERTEX_POINT('',#12374);
#4060=VERTEX_POINT('',#12378);
#4061=VERTEX_POINT('',#12380);
#4062=VERTEX_POINT('',#12386);
#4063=VERTEX_POINT('',#12387);
#4064=VERTEX_POINT('',#12389);
#4065=VERTEX_POINT('',#12391);
#4066=VERTEX_POINT('',#12395);
#4067=VERTEX_POINT('',#12397);
#4068=VERTEX_POINT('',#12401);
#4069=VERTEX_POINT('',#12403);
#4070=VERTEX_POINT('',#12409);
#4071=VERTEX_POINT('',#12410);
#4072=VERTEX_POINT('',#12412);
#4073=VERTEX_POINT('',#12414);
#4074=VERTEX_POINT('',#12418);
#4075=VERTEX_POINT('',#12420);
#4076=VERTEX_POINT('',#12424);
#4077=VERTEX_POINT('',#12426);
#4078=VERTEX_POINT('',#12432);
#4079=VERTEX_POINT('',#12433);
#4080=VERTEX_POINT('',#12435);
#4081=VERTEX_POINT('',#12437);
#4082=VERTEX_POINT('',#12441);
#4083=VERTEX_POINT('',#12443);
#4084=VERTEX_POINT('',#12447);
#4085=VERTEX_POINT('',#12449);
#4086=VERTEX_POINT('',#12455);
#4087=VERTEX_POINT('',#12456);
#4088=VERTEX_POINT('',#12458);
#4089=VERTEX_POINT('',#12460);
#4090=VERTEX_POINT('',#12464);
#4091=VERTEX_POINT('',#12466);
#4092=VERTEX_POINT('',#12470);
#4093=VERTEX_POINT('',#12472);
#4094=VERTEX_POINT('',#12478);
#4095=VERTEX_POINT('',#12479);
#4096=VERTEX_POINT('',#12481);
#4097=VERTEX_POINT('',#12483);
#4098=VERTEX_POINT('',#12487);
#4099=VERTEX_POINT('',#12489);
#4100=VERTEX_POINT('',#12493);
#4101=VERTEX_POINT('',#12495);
#4102=VERTEX_POINT('',#12501);
#4103=VERTEX_POINT('',#12502);
#4104=VERTEX_POINT('',#12504);
#4105=VERTEX_POINT('',#12506);
#4106=VERTEX_POINT('',#12510);
#4107=VERTEX_POINT('',#12512);
#4108=VERTEX_POINT('',#12516);
#4109=VERTEX_POINT('',#12518);
#4110=VERTEX_POINT('',#12524);
#4111=VERTEX_POINT('',#12525);
#4112=VERTEX_POINT('',#12527);
#4113=VERTEX_POINT('',#12529);
#4114=VERTEX_POINT('',#12533);
#4115=VERTEX_POINT('',#12535);
#4116=VERTEX_POINT('',#12539);
#4117=VERTEX_POINT('',#12541);
#4118=VERTEX_POINT('',#12547);
#4119=VERTEX_POINT('',#12548);
#4120=VERTEX_POINT('',#12550);
#4121=VERTEX_POINT('',#12552);
#4122=VERTEX_POINT('',#12556);
#4123=VERTEX_POINT('',#12558);
#4124=VERTEX_POINT('',#12562);
#4125=VERTEX_POINT('',#12564);
#4126=VERTEX_POINT('',#12570);
#4127=VERTEX_POINT('',#12571);
#4128=VERTEX_POINT('',#12573);
#4129=VERTEX_POINT('',#12575);
#4130=VERTEX_POINT('',#12579);
#4131=VERTEX_POINT('',#12581);
#4132=VERTEX_POINT('',#12585);
#4133=VERTEX_POINT('',#12587);
#4134=VERTEX_POINT('',#12593);
#4135=VERTEX_POINT('',#12594);
#4136=VERTEX_POINT('',#12596);
#4137=VERTEX_POINT('',#12598);
#4138=VERTEX_POINT('',#12602);
#4139=VERTEX_POINT('',#12604);
#4140=VERTEX_POINT('',#12608);
#4141=VERTEX_POINT('',#12610);
#4142=VERTEX_POINT('',#12616);
#4143=VERTEX_POINT('',#12617);
#4144=VERTEX_POINT('',#12619);
#4145=VERTEX_POINT('',#12621);
#4146=VERTEX_POINT('',#12625);
#4147=VERTEX_POINT('',#12627);
#4148=VERTEX_POINT('',#12631);
#4149=VERTEX_POINT('',#12633);
#4150=VERTEX_POINT('',#12639);
#4151=VERTEX_POINT('',#12640);
#4152=VERTEX_POINT('',#12642);
#4153=VERTEX_POINT('',#12644);
#4154=VERTEX_POINT('',#12648);
#4155=VERTEX_POINT('',#12650);
#4156=VERTEX_POINT('',#12654);
#4157=VERTEX_POINT('',#12656);
#4158=VERTEX_POINT('',#12662);
#4159=VERTEX_POINT('',#12663);
#4160=VERTEX_POINT('',#12665);
#4161=VERTEX_POINT('',#12667);
#4162=VERTEX_POINT('',#12671);
#4163=VERTEX_POINT('',#12673);
#4164=VERTEX_POINT('',#12677);
#4165=VERTEX_POINT('',#12679);
#4166=VERTEX_POINT('',#12685);
#4167=VERTEX_POINT('',#12686);
#4168=VERTEX_POINT('',#12688);
#4169=VERTEX_POINT('',#12690);
#4170=VERTEX_POINT('',#12694);
#4171=VERTEX_POINT('',#12696);
#4172=VERTEX_POINT('',#12700);
#4173=VERTEX_POINT('',#12702);
#4174=VERTEX_POINT('',#12708);
#4175=VERTEX_POINT('',#12709);
#4176=VERTEX_POINT('',#12711);
#4177=VERTEX_POINT('',#12713);
#4178=VERTEX_POINT('',#12717);
#4179=VERTEX_POINT('',#12719);
#4180=VERTEX_POINT('',#12723);
#4181=VERTEX_POINT('',#12725);
#4182=VERTEX_POINT('',#12731);
#4183=VERTEX_POINT('',#12732);
#4184=VERTEX_POINT('',#12734);
#4185=VERTEX_POINT('',#12736);
#4186=VERTEX_POINT('',#12740);
#4187=VERTEX_POINT('',#12742);
#4188=VERTEX_POINT('',#12746);
#4189=VERTEX_POINT('',#12748);
#4190=VERTEX_POINT('',#12754);
#4191=VERTEX_POINT('',#12755);
#4192=VERTEX_POINT('',#12757);
#4193=VERTEX_POINT('',#12759);
#4194=VERTEX_POINT('',#12763);
#4195=VERTEX_POINT('',#12765);
#4196=VERTEX_POINT('',#12769);
#4197=VERTEX_POINT('',#12771);
#4198=VERTEX_POINT('',#12777);
#4199=VERTEX_POINT('',#12778);
#4200=VERTEX_POINT('',#12780);
#4201=VERTEX_POINT('',#12782);
#4202=VERTEX_POINT('',#12786);
#4203=VERTEX_POINT('',#12788);
#4204=VERTEX_POINT('',#12792);
#4205=VERTEX_POINT('',#12794);
#4206=VERTEX_POINT('',#12800);
#4207=VERTEX_POINT('',#12801);
#4208=VERTEX_POINT('',#12803);
#4209=VERTEX_POINT('',#12805);
#4210=VERTEX_POINT('',#12809);
#4211=VERTEX_POINT('',#12811);
#4212=VERTEX_POINT('',#12815);
#4213=VERTEX_POINT('',#12817);
#4214=VERTEX_POINT('',#12823);
#4215=VERTEX_POINT('',#12824);
#4216=VERTEX_POINT('',#12826);
#4217=VERTEX_POINT('',#12828);
#4218=VERTEX_POINT('',#12832);
#4219=VERTEX_POINT('',#12834);
#4220=VERTEX_POINT('',#12838);
#4221=VERTEX_POINT('',#12840);
#4222=VERTEX_POINT('',#12846);
#4223=VERTEX_POINT('',#12847);
#4224=VERTEX_POINT('',#12849);
#4225=VERTEX_POINT('',#12851);
#4226=VERTEX_POINT('',#12855);
#4227=VERTEX_POINT('',#12857);
#4228=VERTEX_POINT('',#12861);
#4229=VERTEX_POINT('',#12863);
#4230=VERTEX_POINT('',#12869);
#4231=VERTEX_POINT('',#12870);
#4232=VERTEX_POINT('',#12872);
#4233=VERTEX_POINT('',#12874);
#4234=VERTEX_POINT('',#12878);
#4235=VERTEX_POINT('',#12880);
#4236=VERTEX_POINT('',#12884);
#4237=VERTEX_POINT('',#12886);
#4238=VERTEX_POINT('',#12892);
#4239=VERTEX_POINT('',#12893);
#4240=VERTEX_POINT('',#12895);
#4241=VERTEX_POINT('',#12897);
#4242=VERTEX_POINT('',#12901);
#4243=VERTEX_POINT('',#12903);
#4244=VERTEX_POINT('',#12907);
#4245=VERTEX_POINT('',#12909);
#4246=VERTEX_POINT('',#12915);
#4247=VERTEX_POINT('',#12916);
#4248=VERTEX_POINT('',#12918);
#4249=VERTEX_POINT('',#12920);
#4250=VERTEX_POINT('',#12924);
#4251=VERTEX_POINT('',#12926);
#4252=VERTEX_POINT('',#12930);
#4253=VERTEX_POINT('',#12932);
#4254=VERTEX_POINT('',#12939);
#4255=VERTEX_POINT('',#12941);
#4256=VERTEX_POINT('',#12943);
#4257=VERTEX_POINT('',#12945);
#4258=VERTEX_POINT('',#12975);
#4259=VERTEX_POINT('',#12977);
#4260=VERTEX_POINT('',#12980);
#4261=VERTEX_POINT('',#12984);
#4262=VERTEX_POINT('',#12988);
#4263=VERTEX_POINT('',#12989);
#4264=VERTEX_POINT('',#12994);
#4265=VERTEX_POINT('',#12998);
#4810=EDGE_CURVE('',#4022,#4023,#1922,.T.);
#4811=EDGE_CURVE('',#4022,#4024,#1923,.T.);
#4812=EDGE_CURVE('',#4025,#4024,#1924,.T.);
#4813=EDGE_CURVE('',#4023,#4025,#1925,.T.);
#4814=EDGE_CURVE('',#4026,#4022,#1926,.T.);
#4815=EDGE_CURVE('',#4027,#4026,#1927,.T.);
#4816=EDGE_CURVE('',#4024,#4027,#1928,.T.);
#4817=EDGE_CURVE('',#4023,#4028,#1929,.T.);
#4818=EDGE_CURVE('',#4029,#4025,#1930,.T.);
#4819=EDGE_CURVE('',#4028,#4029,#1931,.T.);
#4820=EDGE_CURVE('',#4026,#4028,#1932,.T.);
#4821=EDGE_CURVE('',#4030,#4031,#1933,.T.);
#4822=EDGE_CURVE('',#4030,#4032,#1934,.T.);
#4823=EDGE_CURVE('',#4033,#4032,#1935,.T.);
#4824=EDGE_CURVE('',#4031,#4033,#1936,.T.);
#4825=EDGE_CURVE('',#4034,#4030,#1937,.T.);
#4826=EDGE_CURVE('',#4035,#4034,#1938,.T.);
#4827=EDGE_CURVE('',#4032,#4035,#1939,.T.);
#4828=EDGE_CURVE('',#4031,#4036,#1940,.T.);
#4829=EDGE_CURVE('',#4037,#4033,#1941,.T.);
#4830=EDGE_CURVE('',#4036,#4037,#1942,.T.);
#4831=EDGE_CURVE('',#4034,#4036,#1943,.T.);
#4832=EDGE_CURVE('',#4038,#4039,#1944,.T.);
#4833=EDGE_CURVE('',#4038,#4040,#1945,.T.);
#4834=EDGE_CURVE('',#4041,#4040,#1946,.T.);
#4835=EDGE_CURVE('',#4039,#4041,#1947,.T.);
#4836=EDGE_CURVE('',#4042,#4038,#1948,.T.);
#4837=EDGE_CURVE('',#4043,#4042,#1949,.T.);
#4838=EDGE_CURVE('',#4040,#4043,#1950,.T.);
#4839=EDGE_CURVE('',#4039,#4044,#1951,.T.);
#4840=EDGE_CURVE('',#4045,#4041,#1952,.T.);
#4841=EDGE_CURVE('',#4044,#4045,#1953,.T.);
#4842=EDGE_CURVE('',#4042,#4044,#1954,.T.);
#4843=EDGE_CURVE('',#4046,#4047,#1955,.T.);
#4844=EDGE_CURVE('',#4046,#4048,#1956,.T.);
#4845=EDGE_CURVE('',#4049,#4048,#1957,.T.);
#4846=EDGE_CURVE('',#4047,#4049,#1958,.T.);
#4847=EDGE_CURVE('',#4050,#4046,#1959,.T.);
#4848=EDGE_CURVE('',#4051,#4050,#1960,.T.);
#4849=EDGE_CURVE('',#4048,#4051,#1961,.T.);
#4850=EDGE_CURVE('',#4047,#4052,#1962,.T.);
#4851=EDGE_CURVE('',#4053,#4049,#1963,.T.);
#4852=EDGE_CURVE('',#4052,#4053,#1964,.T.);
#4853=EDGE_CURVE('',#4050,#4052,#1965,.T.);
#4854=EDGE_CURVE('',#4054,#4055,#1966,.T.);
#4855=EDGE_CURVE('',#4054,#4056,#1967,.T.);
#4856=EDGE_CURVE('',#4057,#4056,#1968,.T.);
#4857=EDGE_CURVE('',#4055,#4057,#1969,.T.);
#4858=EDGE_CURVE('',#4058,#4054,#1970,.T.);
#4859=EDGE_CURVE('',#4059,#4058,#1971,.T.);
#4860=EDGE_CURVE('',#4056,#4059,#1972,.T.);
#4861=EDGE_CURVE('',#4055,#4060,#1973,.T.);
#4862=EDGE_CURVE('',#4061,#4057,#1974,.T.);
#4863=EDGE_CURVE('',#4060,#4061,#1975,.T.);
#4864=EDGE_CURVE('',#4058,#4060,#1976,.T.);
#4865=EDGE_CURVE('',#4062,#4063,#1977,.T.);
#4866=EDGE_CURVE('',#4062,#4064,#1978,.T.);
#4867=EDGE_CURVE('',#4065,#4064,#1979,.T.);
#4868=EDGE_CURVE('',#4063,#4065,#1980,.T.);
#4869=EDGE_CURVE('',#4066,#4062,#1981,.T.);
#4870=EDGE_CURVE('',#4067,#4066,#1982,.T.);
#4871=EDGE_CURVE('',#4064,#4067,#1983,.T.);
#4872=EDGE_CURVE('',#4063,#4068,#1984,.T.);
#4873=EDGE_CURVE('',#4069,#4065,#1985,.T.);
#4874=EDGE_CURVE('',#4068,#4069,#1986,.T.);
#4875=EDGE_CURVE('',#4066,#4068,#1987,.T.);
#4876=EDGE_CURVE('',#4070,#4071,#1988,.T.);
#4877=EDGE_CURVE('',#4070,#4072,#1989,.T.);
#4878=EDGE_CURVE('',#4073,#4072,#1990,.T.);
#4879=EDGE_CURVE('',#4071,#4073,#1991,.T.);
#4880=EDGE_CURVE('',#4074,#4070,#1992,.T.);
#4881=EDGE_CURVE('',#4075,#4074,#1993,.T.);
#4882=EDGE_CURVE('',#4072,#4075,#1994,.T.);
#4883=EDGE_CURVE('',#4071,#4076,#1995,.T.);
#4884=EDGE_CURVE('',#4077,#4073,#1996,.T.);
#4885=EDGE_CURVE('',#4076,#4077,#1997,.T.);
#4886=EDGE_CURVE('',#4074,#4076,#1998,.T.);
#4887=EDGE_CURVE('',#4078,#4079,#1999,.T.);
#4888=EDGE_CURVE('',#4078,#4080,#2000,.T.);
#4889=EDGE_CURVE('',#4081,#4080,#2001,.T.);
#4890=EDGE_CURVE('',#4079,#4081,#2002,.T.);
#4891=EDGE_CURVE('',#4082,#4078,#2003,.T.);
#4892=EDGE_CURVE('',#4083,#4082,#2004,.T.);
#4893=EDGE_CURVE('',#4080,#4083,#2005,.T.);
#4894=EDGE_CURVE('',#4079,#4084,#2006,.T.);
#4895=EDGE_CURVE('',#4085,#4081,#2007,.T.);
#4896=EDGE_CURVE('',#4084,#4085,#2008,.T.);
#4897=EDGE_CURVE('',#4082,#4084,#2009,.T.);
#4898=EDGE_CURVE('',#4086,#4087,#2010,.T.);
#4899=EDGE_CURVE('',#4086,#4088,#2011,.T.);
#4900=EDGE_CURVE('',#4089,#4088,#2012,.T.);
#4901=EDGE_CURVE('',#4087,#4089,#2013,.T.);
#4902=EDGE_CURVE('',#4090,#4086,#2014,.T.);
#4903=EDGE_CURVE('',#4091,#4090,#2015,.T.);
#4904=EDGE_CURVE('',#4088,#4091,#2016,.T.);
#4905=EDGE_CURVE('',#4087,#4092,#2017,.T.);
#4906=EDGE_CURVE('',#4093,#4089,#2018,.T.);
#4907=EDGE_CURVE('',#4092,#4093,#2019,.T.);
#4908=EDGE_CURVE('',#4090,#4092,#2020,.T.);
#4909=EDGE_CURVE('',#4094,#4095,#2021,.T.);
#4910=EDGE_CURVE('',#4094,#4096,#2022,.T.);
#4911=EDGE_CURVE('',#4097,#4096,#2023,.T.);
#4912=EDGE_CURVE('',#4095,#4097,#2024,.T.);
#4913=EDGE_CURVE('',#4098,#4094,#2025,.T.);
#4914=EDGE_CURVE('',#4099,#4098,#2026,.T.);
#4915=EDGE_CURVE('',#4096,#4099,#2027,.T.);
#4916=EDGE_CURVE('',#4095,#4100,#2028,.T.);
#4917=EDGE_CURVE('',#4101,#4097,#2029,.T.);
#4918=EDGE_CURVE('',#4100,#4101,#2030,.T.);
#4919=EDGE_CURVE('',#4098,#4100,#2031,.T.);
#4920=EDGE_CURVE('',#4102,#4103,#2032,.T.);
#4921=EDGE_CURVE('',#4102,#4104,#2033,.T.);
#4922=EDGE_CURVE('',#4105,#4104,#2034,.T.);
#4923=EDGE_CURVE('',#4103,#4105,#2035,.T.);
#4924=EDGE_CURVE('',#4106,#4102,#2036,.T.);
#4925=EDGE_CURVE('',#4107,#4106,#2037,.T.);
#4926=EDGE_CURVE('',#4104,#4107,#2038,.T.);
#4927=EDGE_CURVE('',#4103,#4108,#2039,.T.);
#4928=EDGE_CURVE('',#4109,#4105,#2040,.T.);
#4929=EDGE_CURVE('',#4108,#4109,#2041,.T.);
#4930=EDGE_CURVE('',#4106,#4108,#2042,.T.);
#4931=EDGE_CURVE('',#4110,#4111,#2043,.T.);
#4932=EDGE_CURVE('',#4110,#4112,#2044,.T.);
#4933=EDGE_CURVE('',#4113,#4112,#2045,.T.);
#4934=EDGE_CURVE('',#4111,#4113,#2046,.T.);
#4935=EDGE_CURVE('',#4114,#4110,#2047,.T.);
#4936=EDGE_CURVE('',#4115,#4114,#2048,.T.);
#4937=EDGE_CURVE('',#4112,#4115,#2049,.T.);
#4938=EDGE_CURVE('',#4111,#4116,#2050,.T.);
#4939=EDGE_CURVE('',#4117,#4113,#2051,.T.);
#4940=EDGE_CURVE('',#4116,#4117,#2052,.T.);
#4941=EDGE_CURVE('',#4114,#4116,#2053,.T.);
#4942=EDGE_CURVE('',#4118,#4119,#2054,.T.);
#4943=EDGE_CURVE('',#4118,#4120,#2055,.T.);
#4944=EDGE_CURVE('',#4121,#4120,#2056,.T.);
#4945=EDGE_CURVE('',#4119,#4121,#2057,.T.);
#4946=EDGE_CURVE('',#4122,#4118,#2058,.T.);
#4947=EDGE_CURVE('',#4123,#4122,#2059,.T.);
#4948=EDGE_CURVE('',#4120,#4123,#2060,.T.);
#4949=EDGE_CURVE('',#4119,#4124,#2061,.T.);
#4950=EDGE_CURVE('',#4125,#4121,#2062,.T.);
#4951=EDGE_CURVE('',#4124,#4125,#2063,.T.);
#4952=EDGE_CURVE('',#4122,#4124,#2064,.T.);
#4953=EDGE_CURVE('',#4126,#4127,#2065,.T.);
#4954=EDGE_CURVE('',#4126,#4128,#2066,.T.);
#4955=EDGE_CURVE('',#4129,#4128,#2067,.T.);
#4956=EDGE_CURVE('',#4127,#4129,#2068,.T.);
#4957=EDGE_CURVE('',#4130,#4126,#2069,.T.);
#4958=EDGE_CURVE('',#4131,#4130,#2070,.T.);
#4959=EDGE_CURVE('',#4128,#4131,#2071,.T.);
#4960=EDGE_CURVE('',#4127,#4132,#2072,.T.);
#4961=EDGE_CURVE('',#4133,#4129,#2073,.T.);
#4962=EDGE_CURVE('',#4132,#4133,#2074,.T.);
#4963=EDGE_CURVE('',#4130,#4132,#2075,.T.);
#4964=EDGE_CURVE('',#4134,#4135,#2076,.T.);
#4965=EDGE_CURVE('',#4134,#4136,#2077,.T.);
#4966=EDGE_CURVE('',#4137,#4136,#2078,.T.);
#4967=EDGE_CURVE('',#4135,#4137,#2079,.T.);
#4968=EDGE_CURVE('',#4138,#4134,#2080,.T.);
#4969=EDGE_CURVE('',#4139,#4138,#2081,.T.);
#4970=EDGE_CURVE('',#4136,#4139,#2082,.T.);
#4971=EDGE_CURVE('',#4135,#4140,#2083,.T.);
#4972=EDGE_CURVE('',#4141,#4137,#2084,.T.);
#4973=EDGE_CURVE('',#4140,#4141,#2085,.T.);
#4974=EDGE_CURVE('',#4138,#4140,#2086,.T.);
#4975=EDGE_CURVE('',#4142,#4143,#2087,.T.);
#4976=EDGE_CURVE('',#4142,#4144,#2088,.T.);
#4977=EDGE_CURVE('',#4145,#4144,#2089,.T.);
#4978=EDGE_CURVE('',#4143,#4145,#2090,.T.);
#4979=EDGE_CURVE('',#4146,#4142,#2091,.T.);
#4980=EDGE_CURVE('',#4147,#4146,#2092,.T.);
#4981=EDGE_CURVE('',#4144,#4147,#2093,.T.);
#4982=EDGE_CURVE('',#4143,#4148,#2094,.T.);
#4983=EDGE_CURVE('',#4149,#4145,#2095,.T.);
#4984=EDGE_CURVE('',#4148,#4149,#2096,.T.);
#4985=EDGE_CURVE('',#4146,#4148,#2097,.T.);
#4986=EDGE_CURVE('',#4150,#4151,#2098,.T.);
#4987=EDGE_CURVE('',#4150,#4152,#2099,.T.);
#4988=EDGE_CURVE('',#4153,#4152,#2100,.T.);
#4989=EDGE_CURVE('',#4151,#4153,#2101,.T.);
#4990=EDGE_CURVE('',#4154,#4150,#2102,.T.);
#4991=EDGE_CURVE('',#4155,#4154,#2103,.T.);
#4992=EDGE_CURVE('',#4152,#4155,#2104,.T.);
#4993=EDGE_CURVE('',#4151,#4156,#2105,.T.);
#4994=EDGE_CURVE('',#4157,#4153,#2106,.T.);
#4995=EDGE_CURVE('',#4156,#4157,#2107,.T.);
#4996=EDGE_CURVE('',#4154,#4156,#2108,.T.);
#4997=EDGE_CURVE('',#4158,#4159,#2109,.T.);
#4998=EDGE_CURVE('',#4158,#4160,#2110,.T.);
#4999=EDGE_CURVE('',#4161,#4160,#2111,.T.);
#5000=EDGE_CURVE('',#4159,#4161,#2112,.T.);
#5001=EDGE_CURVE('',#4162,#4158,#2113,.T.);
#5002=EDGE_CURVE('',#4163,#4162,#2114,.T.);
#5003=EDGE_CURVE('',#4160,#4163,#2115,.T.);
#5004=EDGE_CURVE('',#4159,#4164,#2116,.T.);
#5005=EDGE_CURVE('',#4165,#4161,#2117,.T.);
#5006=EDGE_CURVE('',#4164,#4165,#2118,.T.);
#5007=EDGE_CURVE('',#4162,#4164,#2119,.T.);
#5008=EDGE_CURVE('',#4166,#4167,#2120,.T.);
#5009=EDGE_CURVE('',#4166,#4168,#2121,.T.);
#5010=EDGE_CURVE('',#4169,#4168,#2122,.T.);
#5011=EDGE_CURVE('',#4167,#4169,#2123,.T.);
#5012=EDGE_CURVE('',#4170,#4166,#2124,.T.);
#5013=EDGE_CURVE('',#4171,#4170,#2125,.T.);
#5014=EDGE_CURVE('',#4168,#4171,#2126,.T.);
#5015=EDGE_CURVE('',#4167,#4172,#2127,.T.);
#5016=EDGE_CURVE('',#4173,#4169,#2128,.T.);
#5017=EDGE_CURVE('',#4172,#4173,#2129,.T.);
#5018=EDGE_CURVE('',#4170,#4172,#2130,.T.);
#5019=EDGE_CURVE('',#4174,#4175,#2131,.T.);
#5020=EDGE_CURVE('',#4174,#4176,#2132,.T.);
#5021=EDGE_CURVE('',#4177,#4176,#2133,.T.);
#5022=EDGE_CURVE('',#4175,#4177,#2134,.T.);
#5023=EDGE_CURVE('',#4178,#4174,#2135,.T.);
#5024=EDGE_CURVE('',#4179,#4178,#2136,.T.);
#5025=EDGE_CURVE('',#4176,#4179,#2137,.T.);
#5026=EDGE_CURVE('',#4175,#4180,#2138,.T.);
#5027=EDGE_CURVE('',#4181,#4177,#2139,.T.);
#5028=EDGE_CURVE('',#4180,#4181,#2140,.T.);
#5029=EDGE_CURVE('',#4178,#4180,#2141,.T.);
#5030=EDGE_CURVE('',#4182,#4183,#2142,.T.);
#5031=EDGE_CURVE('',#4182,#4184,#2143,.T.);
#5032=EDGE_CURVE('',#4185,#4184,#2144,.T.);
#5033=EDGE_CURVE('',#4183,#4185,#2145,.T.);
#5034=EDGE_CURVE('',#4186,#4182,#2146,.T.);
#5035=EDGE_CURVE('',#4187,#4186,#2147,.T.);
#5036=EDGE_CURVE('',#4184,#4187,#2148,.T.);
#5037=EDGE_CURVE('',#4183,#4188,#2149,.T.);
#5038=EDGE_CURVE('',#4189,#4185,#2150,.T.);
#5039=EDGE_CURVE('',#4188,#4189,#2151,.T.);
#5040=EDGE_CURVE('',#4186,#4188,#2152,.T.);
#5041=EDGE_CURVE('',#4190,#4191,#2153,.T.);
#5042=EDGE_CURVE('',#4190,#4192,#2154,.T.);
#5043=EDGE_CURVE('',#4193,#4192,#2155,.T.);
#5044=EDGE_CURVE('',#4191,#4193,#2156,.T.);
#5045=EDGE_CURVE('',#4194,#4190,#2157,.T.);
#5046=EDGE_CURVE('',#4195,#4194,#2158,.T.);
#5047=EDGE_CURVE('',#4192,#4195,#2159,.T.);
#5048=EDGE_CURVE('',#4191,#4196,#2160,.T.);
#5049=EDGE_CURVE('',#4197,#4193,#2161,.T.);
#5050=EDGE_CURVE('',#4196,#4197,#2162,.T.);
#5051=EDGE_CURVE('',#4194,#4196,#2163,.T.);
#5052=EDGE_CURVE('',#4198,#4199,#2164,.T.);
#5053=EDGE_CURVE('',#4198,#4200,#2165,.T.);
#5054=EDGE_CURVE('',#4201,#4200,#2166,.T.);
#5055=EDGE_CURVE('',#4199,#4201,#2167,.T.);
#5056=EDGE_CURVE('',#4202,#4198,#2168,.T.);
#5057=EDGE_CURVE('',#4203,#4202,#2169,.T.);
#5058=EDGE_CURVE('',#4200,#4203,#2170,.T.);
#5059=EDGE_CURVE('',#4199,#4204,#2171,.T.);
#5060=EDGE_CURVE('',#4205,#4201,#2172,.T.);
#5061=EDGE_CURVE('',#4204,#4205,#2173,.T.);
#5062=EDGE_CURVE('',#4202,#4204,#2174,.T.);
#5063=EDGE_CURVE('',#4206,#4207,#2175,.T.);
#5064=EDGE_CURVE('',#4206,#4208,#2176,.T.);
#5065=EDGE_CURVE('',#4209,#4208,#2177,.T.);
#5066=EDGE_CURVE('',#4207,#4209,#2178,.T.);
#5067=EDGE_CURVE('',#4210,#4206,#2179,.T.);
#5068=EDGE_CURVE('',#4211,#4210,#2180,.T.);
#5069=EDGE_CURVE('',#4208,#4211,#2181,.T.);
#5070=EDGE_CURVE('',#4207,#4212,#2182,.T.);
#5071=EDGE_CURVE('',#4213,#4209,#2183,.T.);
#5072=EDGE_CURVE('',#4212,#4213,#2184,.T.);
#5073=EDGE_CURVE('',#4210,#4212,#2185,.T.);
#5074=EDGE_CURVE('',#4214,#4215,#2186,.T.);
#5075=EDGE_CURVE('',#4214,#4216,#2187,.T.);
#5076=EDGE_CURVE('',#4217,#4216,#2188,.T.);
#5077=EDGE_CURVE('',#4215,#4217,#2189,.T.);
#5078=EDGE_CURVE('',#4218,#4214,#2190,.T.);
#5079=EDGE_CURVE('',#4219,#4218,#2191,.T.);
#5080=EDGE_CURVE('',#4216,#4219,#2192,.T.);
#5081=EDGE_CURVE('',#4215,#4220,#2193,.T.);
#5082=EDGE_CURVE('',#4221,#4217,#2194,.T.);
#5083=EDGE_CURVE('',#4220,#4221,#2195,.T.);
#5084=EDGE_CURVE('',#4218,#4220,#2196,.T.);
#5085=EDGE_CURVE('',#4222,#4223,#2197,.T.);
#5086=EDGE_CURVE('',#4222,#4224,#2198,.T.);
#5087=EDGE_CURVE('',#4225,#4224,#2199,.T.);
#5088=EDGE_CURVE('',#4223,#4225,#2200,.T.);
#5089=EDGE_CURVE('',#4226,#4222,#2201,.T.);
#5090=EDGE_CURVE('',#4227,#4226,#2202,.T.);
#5091=EDGE_CURVE('',#4224,#4227,#2203,.T.);
#5092=EDGE_CURVE('',#4223,#4228,#2204,.T.);
#5093=EDGE_CURVE('',#4229,#4225,#2205,.T.);
#5094=EDGE_CURVE('',#4228,#4229,#2206,.T.);
#5095=EDGE_CURVE('',#4226,#4228,#2207,.T.);
#5096=EDGE_CURVE('',#4230,#4231,#2208,.T.);
#5097=EDGE_CURVE('',#4230,#4232,#2209,.T.);
#5098=EDGE_CURVE('',#4233,#4232,#2210,.T.);
#5099=EDGE_CURVE('',#4231,#4233,#2211,.T.);
#5100=EDGE_CURVE('',#4234,#4230,#2212,.T.);
#5101=EDGE_CURVE('',#4235,#4234,#2213,.T.);
#5102=EDGE_CURVE('',#4232,#4235,#2214,.T.);
#5103=EDGE_CURVE('',#4231,#4236,#2215,.T.);
#5104=EDGE_CURVE('',#4237,#4233,#2216,.T.);
#5105=EDGE_CURVE('',#4236,#4237,#2217,.T.);
#5106=EDGE_CURVE('',#4234,#4236,#2218,.T.);
#5107=EDGE_CURVE('',#4238,#4239,#2219,.T.);
#5108=EDGE_CURVE('',#4238,#4240,#2220,.T.);
#5109=EDGE_CURVE('',#4241,#4240,#2221,.T.);
#5110=EDGE_CURVE('',#4239,#4241,#2222,.T.);
#5111=EDGE_CURVE('',#4242,#4238,#2223,.T.);
#5112=EDGE_CURVE('',#4243,#4242,#2224,.T.);
#5113=EDGE_CURVE('',#4240,#4243,#2225,.T.);
#5114=EDGE_CURVE('',#4239,#4244,#2226,.T.);
#5115=EDGE_CURVE('',#4245,#4241,#2227,.T.);
#5116=EDGE_CURVE('',#4244,#4245,#2228,.T.);
#5117=EDGE_CURVE('',#4242,#4244,#2229,.T.);
#5118=EDGE_CURVE('',#4246,#4247,#2230,.T.);
#5119=EDGE_CURVE('',#4246,#4248,#2231,.T.);
#5120=EDGE_CURVE('',#4249,#4248,#2232,.T.);
#5121=EDGE_CURVE('',#4247,#4249,#2233,.T.);
#5122=EDGE_CURVE('',#4250,#4246,#2234,.T.);
#5123=EDGE_CURVE('',#4251,#4250,#2235,.T.);
#5124=EDGE_CURVE('',#4248,#4251,#2236,.T.);
#5125=EDGE_CURVE('',#4247,#4252,#2237,.T.);
#5126=EDGE_CURVE('',#4253,#4249,#2238,.T.);
#5127=EDGE_CURVE('',#4252,#4253,#2239,.T.);
#5128=EDGE_CURVE('',#4250,#4252,#2240,.T.);
#5129=EDGE_CURVE('',#4027,#4253,#2241,.T.);
#5130=EDGE_CURVE('',#4251,#4254,#2242,.T.);
#5131=EDGE_CURVE('',#4254,#4255,#2243,.T.);
#5132=EDGE_CURVE('',#4255,#4256,#2244,.T.);
#5133=EDGE_CURVE('',#4256,#4257,#2245,.T.);
#5134=EDGE_CURVE('',#4257,#4197,#2246,.T.);
#5135=EDGE_CURVE('',#4195,#4141,#2247,.T.);
#5136=EDGE_CURVE('',#4139,#4133,#2248,.T.);
#5137=EDGE_CURVE('',#4131,#4149,#2249,.T.);
#5138=EDGE_CURVE('',#4147,#4125,#2250,.T.);
#5139=EDGE_CURVE('',#4123,#4157,#2251,.T.);
#5140=EDGE_CURVE('',#4155,#4117,#2252,.T.);
#5141=EDGE_CURVE('',#4115,#4165,#2253,.T.);
#5142=EDGE_CURVE('',#4163,#4109,#2254,.T.);
#5143=EDGE_CURVE('',#4107,#4173,#2255,.T.);
#5144=EDGE_CURVE('',#4171,#4101,#2256,.T.);
#5145=EDGE_CURVE('',#4099,#4181,#2257,.T.);
#5146=EDGE_CURVE('',#4179,#4093,#2258,.T.);
#5147=EDGE_CURVE('',#4091,#4189,#2259,.T.);
#5148=EDGE_CURVE('',#4187,#4085,#2260,.T.);
#5149=EDGE_CURVE('',#4083,#4077,#2261,.T.);
#5150=EDGE_CURVE('',#4075,#4205,#2262,.T.);
#5151=EDGE_CURVE('',#4203,#4069,#2263,.T.);
#5152=EDGE_CURVE('',#4067,#4213,#2264,.T.);
#5153=EDGE_CURVE('',#4211,#4061,#2265,.T.);
#5154=EDGE_CURVE('',#4059,#4221,#2266,.T.);
#5155=EDGE_CURVE('',#4219,#4053,#2267,.T.);
#5156=EDGE_CURVE('',#4051,#4229,#2268,.T.);
#5157=EDGE_CURVE('',#4227,#4045,#2269,.T.);
#5158=EDGE_CURVE('',#4043,#4237,#2270,.T.);
#5159=EDGE_CURVE('',#4235,#4037,#2271,.T.);
#5160=EDGE_CURVE('',#4035,#4245,#2272,.T.);
#5161=EDGE_CURVE('',#4243,#4029,#2273,.T.);
#5162=EDGE_CURVE('',#4258,#4258,#3826,.T.);
#5163=EDGE_CURVE('',#4259,#4259,#3827,.T.);
#5164=EDGE_CURVE('',#4260,#4260,#3828,.T.);
#5165=EDGE_CURVE('',#4260,#4259,#2274,.T.);
#5166=EDGE_CURVE('',#4261,#4261,#3829,.T.);
#5167=EDGE_CURVE('',#4261,#4258,#2275,.T.);
#5168=EDGE_CURVE('',#4262,#4263,#2276,.T.);
#5169=EDGE_CURVE('',#4263,#4256,#2277,.T.);
#5170=EDGE_CURVE('',#4262,#4255,#2278,.T.);
#5171=EDGE_CURVE('',#4264,#4262,#2279,.T.);
#5172=EDGE_CURVE('',#4264,#4254,#2280,.T.);
#5173=EDGE_CURVE('',#4265,#4257,#2281,.T.);
#5174=EDGE_CURVE('',#4265,#4264,#2282,.T.);
#5175=EDGE_CURVE('',#4263,#4265,#2283,.T.);
#6065=ORIENTED_EDGE('',*,*,#4810,.F.);
#6066=ORIENTED_EDGE('',*,*,#4811,.T.);
#6067=ORIENTED_EDGE('',*,*,#4812,.F.);
#6068=ORIENTED_EDGE('',*,*,#4813,.F.);
#6069=ORIENTED_EDGE('',*,*,#4814,.F.);
#6070=ORIENTED_EDGE('',*,*,#4815,.F.);
#6071=ORIENTED_EDGE('',*,*,#4816,.F.);
#6072=ORIENTED_EDGE('',*,*,#4811,.F.);
#6073=ORIENTED_EDGE('',*,*,#4817,.F.);
#6074=ORIENTED_EDGE('',*,*,#4813,.T.);
#6075=ORIENTED_EDGE('',*,*,#4818,.F.);
#6076=ORIENTED_EDGE('',*,*,#4819,.F.);
#6077=ORIENTED_EDGE('',*,*,#4817,.T.);
#6078=ORIENTED_EDGE('',*,*,#4820,.F.);
#6079=ORIENTED_EDGE('',*,*,#4814,.T.);
#6080=ORIENTED_EDGE('',*,*,#4810,.T.);
#6081=ORIENTED_EDGE('',*,*,#4821,.F.);
#6082=ORIENTED_EDGE('',*,*,#4822,.T.);
#6083=ORIENTED_EDGE('',*,*,#4823,.F.);
#6084=ORIENTED_EDGE('',*,*,#4824,.F.);
#6085=ORIENTED_EDGE('',*,*,#4825,.F.);
#6086=ORIENTED_EDGE('',*,*,#4826,.F.);
#6087=ORIENTED_EDGE('',*,*,#4827,.F.);
#6088=ORIENTED_EDGE('',*,*,#4822,.F.);
#6089=ORIENTED_EDGE('',*,*,#4828,.F.);
#6090=ORIENTED_EDGE('',*,*,#4824,.T.);
#6091=ORIENTED_EDGE('',*,*,#4829,.F.);
#6092=ORIENTED_EDGE('',*,*,#4830,.F.);
#6093=ORIENTED_EDGE('',*,*,#4828,.T.);
#6094=ORIENTED_EDGE('',*,*,#4831,.F.);
#6095=ORIENTED_EDGE('',*,*,#4825,.T.);
#6096=ORIENTED_EDGE('',*,*,#4821,.T.);
#6097=ORIENTED_EDGE('',*,*,#4832,.F.);
#6098=ORIENTED_EDGE('',*,*,#4833,.T.);
#6099=ORIENTED_EDGE('',*,*,#4834,.F.);
#6100=ORIENTED_EDGE('',*,*,#4835,.F.);
#6101=ORIENTED_EDGE('',*,*,#4836,.F.);
#6102=ORIENTED_EDGE('',*,*,#4837,.F.);
#6103=ORIENTED_EDGE('',*,*,#4838,.F.);
#6104=ORIENTED_EDGE('',*,*,#4833,.F.);
#6105=ORIENTED_EDGE('',*,*,#4839,.F.);
#6106=ORIENTED_EDGE('',*,*,#4835,.T.);
#6107=ORIENTED_EDGE('',*,*,#4840,.F.);
#6108=ORIENTED_EDGE('',*,*,#4841,.F.);
#6109=ORIENTED_EDGE('',*,*,#4839,.T.);
#6110=ORIENTED_EDGE('',*,*,#4842,.F.);
#6111=ORIENTED_EDGE('',*,*,#4836,.T.);
#6112=ORIENTED_EDGE('',*,*,#4832,.T.);
#6113=ORIENTED_EDGE('',*,*,#4843,.F.);
#6114=ORIENTED_EDGE('',*,*,#4844,.T.);
#6115=ORIENTED_EDGE('',*,*,#4845,.F.);
#6116=ORIENTED_EDGE('',*,*,#4846,.F.);
#6117=ORIENTED_EDGE('',*,*,#4847,.F.);
#6118=ORIENTED_EDGE('',*,*,#4848,.F.);
#6119=ORIENTED_EDGE('',*,*,#4849,.F.);
#6120=ORIENTED_EDGE('',*,*,#4844,.F.);
#6121=ORIENTED_EDGE('',*,*,#4850,.F.);
#6122=ORIENTED_EDGE('',*,*,#4846,.T.);
#6123=ORIENTED_EDGE('',*,*,#4851,.F.);
#6124=ORIENTED_EDGE('',*,*,#4852,.F.);
#6125=ORIENTED_EDGE('',*,*,#4850,.T.);
#6126=ORIENTED_EDGE('',*,*,#4853,.F.);
#6127=ORIENTED_EDGE('',*,*,#4847,.T.);
#6128=ORIENTED_EDGE('',*,*,#4843,.T.);
#6129=ORIENTED_EDGE('',*,*,#4854,.F.);
#6130=ORIENTED_EDGE('',*,*,#4855,.T.);
#6131=ORIENTED_EDGE('',*,*,#4856,.F.);
#6132=ORIENTED_EDGE('',*,*,#4857,.F.);
#6133=ORIENTED_EDGE('',*,*,#4858,.F.);
#6134=ORIENTED_EDGE('',*,*,#4859,.F.);
#6135=ORIENTED_EDGE('',*,*,#4860,.F.);
#6136=ORIENTED_EDGE('',*,*,#4855,.F.);
#6137=ORIENTED_EDGE('',*,*,#4861,.F.);
#6138=ORIENTED_EDGE('',*,*,#4857,.T.);
#6139=ORIENTED_EDGE('',*,*,#4862,.F.);
#6140=ORIENTED_EDGE('',*,*,#4863,.F.);
#6141=ORIENTED_EDGE('',*,*,#4861,.T.);
#6142=ORIENTED_EDGE('',*,*,#4864,.F.);
#6143=ORIENTED_EDGE('',*,*,#4858,.T.);
#6144=ORIENTED_EDGE('',*,*,#4854,.T.);
#6145=ORIENTED_EDGE('',*,*,#4865,.F.);
#6146=ORIENTED_EDGE('',*,*,#4866,.T.);
#6147=ORIENTED_EDGE('',*,*,#4867,.F.);
#6148=ORIENTED_EDGE('',*,*,#4868,.F.);
#6149=ORIENTED_EDGE('',*,*,#4869,.F.);
#6150=ORIENTED_EDGE('',*,*,#4870,.F.);
#6151=ORIENTED_EDGE('',*,*,#4871,.F.);
#6152=ORIENTED_EDGE('',*,*,#4866,.F.);
#6153=ORIENTED_EDGE('',*,*,#4872,.F.);
#6154=ORIENTED_EDGE('',*,*,#4868,.T.);
#6155=ORIENTED_EDGE('',*,*,#4873,.F.);
#6156=ORIENTED_EDGE('',*,*,#4874,.F.);
#6157=ORIENTED_EDGE('',*,*,#4872,.T.);
#6158=ORIENTED_EDGE('',*,*,#4875,.F.);
#6159=ORIENTED_EDGE('',*,*,#4869,.T.);
#6160=ORIENTED_EDGE('',*,*,#4865,.T.);
#6161=ORIENTED_EDGE('',*,*,#4876,.F.);
#6162=ORIENTED_EDGE('',*,*,#4877,.T.);
#6163=ORIENTED_EDGE('',*,*,#4878,.F.);
#6164=ORIENTED_EDGE('',*,*,#4879,.F.);
#6165=ORIENTED_EDGE('',*,*,#4880,.F.);
#6166=ORIENTED_EDGE('',*,*,#4881,.F.);
#6167=ORIENTED_EDGE('',*,*,#4882,.F.);
#6168=ORIENTED_EDGE('',*,*,#4877,.F.);
#6169=ORIENTED_EDGE('',*,*,#4883,.F.);
#6170=ORIENTED_EDGE('',*,*,#4879,.T.);
#6171=ORIENTED_EDGE('',*,*,#4884,.F.);
#6172=ORIENTED_EDGE('',*,*,#4885,.F.);
#6173=ORIENTED_EDGE('',*,*,#4883,.T.);
#6174=ORIENTED_EDGE('',*,*,#4886,.F.);
#6175=ORIENTED_EDGE('',*,*,#4880,.T.);
#6176=ORIENTED_EDGE('',*,*,#4876,.T.);
#6177=ORIENTED_EDGE('',*,*,#4887,.F.);
#6178=ORIENTED_EDGE('',*,*,#4888,.T.);
#6179=ORIENTED_EDGE('',*,*,#4889,.F.);
#6180=ORIENTED_EDGE('',*,*,#4890,.F.);
#6181=ORIENTED_EDGE('',*,*,#4891,.F.);
#6182=ORIENTED_EDGE('',*,*,#4892,.F.);
#6183=ORIENTED_EDGE('',*,*,#4893,.F.);
#6184=ORIENTED_EDGE('',*,*,#4888,.F.);
#6185=ORIENTED_EDGE('',*,*,#4894,.F.);
#6186=ORIENTED_EDGE('',*,*,#4890,.T.);
#6187=ORIENTED_EDGE('',*,*,#4895,.F.);
#6188=ORIENTED_EDGE('',*,*,#4896,.F.);
#6189=ORIENTED_EDGE('',*,*,#4894,.T.);
#6190=ORIENTED_EDGE('',*,*,#4897,.F.);
#6191=ORIENTED_EDGE('',*,*,#4891,.T.);
#6192=ORIENTED_EDGE('',*,*,#4887,.T.);
#6193=ORIENTED_EDGE('',*,*,#4898,.F.);
#6194=ORIENTED_EDGE('',*,*,#4899,.T.);
#6195=ORIENTED_EDGE('',*,*,#4900,.F.);
#6196=ORIENTED_EDGE('',*,*,#4901,.F.);
#6197=ORIENTED_EDGE('',*,*,#4902,.F.);
#6198=ORIENTED_EDGE('',*,*,#4903,.F.);
#6199=ORIENTED_EDGE('',*,*,#4904,.F.);
#6200=ORIENTED_EDGE('',*,*,#4899,.F.);
#6201=ORIENTED_EDGE('',*,*,#4905,.F.);
#6202=ORIENTED_EDGE('',*,*,#4901,.T.);
#6203=ORIENTED_EDGE('',*,*,#4906,.F.);
#6204=ORIENTED_EDGE('',*,*,#4907,.F.);
#6205=ORIENTED_EDGE('',*,*,#4905,.T.);
#6206=ORIENTED_EDGE('',*,*,#4908,.F.);
#6207=ORIENTED_EDGE('',*,*,#4902,.T.);
#6208=ORIENTED_EDGE('',*,*,#4898,.T.);
#6209=ORIENTED_EDGE('',*,*,#4909,.F.);
#6210=ORIENTED_EDGE('',*,*,#4910,.T.);
#6211=ORIENTED_EDGE('',*,*,#4911,.F.);
#6212=ORIENTED_EDGE('',*,*,#4912,.F.);
#6213=ORIENTED_EDGE('',*,*,#4913,.F.);
#6214=ORIENTED_EDGE('',*,*,#4914,.F.);
#6215=ORIENTED_EDGE('',*,*,#4915,.F.);
#6216=ORIENTED_EDGE('',*,*,#4910,.F.);
#6217=ORIENTED_EDGE('',*,*,#4916,.F.);
#6218=ORIENTED_EDGE('',*,*,#4912,.T.);
#6219=ORIENTED_EDGE('',*,*,#4917,.F.);
#6220=ORIENTED_EDGE('',*,*,#4918,.F.);
#6221=ORIENTED_EDGE('',*,*,#4916,.T.);
#6222=ORIENTED_EDGE('',*,*,#4919,.F.);
#6223=ORIENTED_EDGE('',*,*,#4913,.T.);
#6224=ORIENTED_EDGE('',*,*,#4909,.T.);
#6225=ORIENTED_EDGE('',*,*,#4920,.F.);
#6226=ORIENTED_EDGE('',*,*,#4921,.T.);
#6227=ORIENTED_EDGE('',*,*,#4922,.F.);
#6228=ORIENTED_EDGE('',*,*,#4923,.F.);
#6229=ORIENTED_EDGE('',*,*,#4924,.F.);
#6230=ORIENTED_EDGE('',*,*,#4925,.F.);
#6231=ORIENTED_EDGE('',*,*,#4926,.F.);
#6232=ORIENTED_EDGE('',*,*,#4921,.F.);
#6233=ORIENTED_EDGE('',*,*,#4927,.F.);
#6234=ORIENTED_EDGE('',*,*,#4923,.T.);
#6235=ORIENTED_EDGE('',*,*,#4928,.F.);
#6236=ORIENTED_EDGE('',*,*,#4929,.F.);
#6237=ORIENTED_EDGE('',*,*,#4927,.T.);
#6238=ORIENTED_EDGE('',*,*,#4930,.F.);
#6239=ORIENTED_EDGE('',*,*,#4924,.T.);
#6240=ORIENTED_EDGE('',*,*,#4920,.T.);
#6241=ORIENTED_EDGE('',*,*,#4931,.F.);
#6242=ORIENTED_EDGE('',*,*,#4932,.T.);
#6243=ORIENTED_EDGE('',*,*,#4933,.F.);
#6244=ORIENTED_EDGE('',*,*,#4934,.F.);
#6245=ORIENTED_EDGE('',*,*,#4935,.F.);
#6246=ORIENTED_EDGE('',*,*,#4936,.F.);
#6247=ORIENTED_EDGE('',*,*,#4937,.F.);
#6248=ORIENTED_EDGE('',*,*,#4932,.F.);
#6249=ORIENTED_EDGE('',*,*,#4938,.F.);
#6250=ORIENTED_EDGE('',*,*,#4934,.T.);
#6251=ORIENTED_EDGE('',*,*,#4939,.F.);
#6252=ORIENTED_EDGE('',*,*,#4940,.F.);
#6253=ORIENTED_EDGE('',*,*,#4938,.T.);
#6254=ORIENTED_EDGE('',*,*,#4941,.F.);
#6255=ORIENTED_EDGE('',*,*,#4935,.T.);
#6256=ORIENTED_EDGE('',*,*,#4931,.T.);
#6257=ORIENTED_EDGE('',*,*,#4942,.F.);
#6258=ORIENTED_EDGE('',*,*,#4943,.T.);
#6259=ORIENTED_EDGE('',*,*,#4944,.F.);
#6260=ORIENTED_EDGE('',*,*,#4945,.F.);
#6261=ORIENTED_EDGE('',*,*,#4946,.F.);
#6262=ORIENTED_EDGE('',*,*,#4947,.F.);
#6263=ORIENTED_EDGE('',*,*,#4948,.F.);
#6264=ORIENTED_EDGE('',*,*,#4943,.F.);
#6265=ORIENTED_EDGE('',*,*,#4949,.F.);
#6266=ORIENTED_EDGE('',*,*,#4945,.T.);
#6267=ORIENTED_EDGE('',*,*,#4950,.F.);
#6268=ORIENTED_EDGE('',*,*,#4951,.F.);
#6269=ORIENTED_EDGE('',*,*,#4949,.T.);
#6270=ORIENTED_EDGE('',*,*,#4952,.F.);
#6271=ORIENTED_EDGE('',*,*,#4946,.T.);
#6272=ORIENTED_EDGE('',*,*,#4942,.T.);
#6273=ORIENTED_EDGE('',*,*,#4953,.F.);
#6274=ORIENTED_EDGE('',*,*,#4954,.T.);
#6275=ORIENTED_EDGE('',*,*,#4955,.F.);
#6276=ORIENTED_EDGE('',*,*,#4956,.F.);
#6277=ORIENTED_EDGE('',*,*,#4957,.F.);
#6278=ORIENTED_EDGE('',*,*,#4958,.F.);
#6279=ORIENTED_EDGE('',*,*,#4959,.F.);
#6280=ORIENTED_EDGE('',*,*,#4954,.F.);
#6281=ORIENTED_EDGE('',*,*,#4960,.F.);
#6282=ORIENTED_EDGE('',*,*,#4956,.T.);
#6283=ORIENTED_EDGE('',*,*,#4961,.F.);
#6284=ORIENTED_EDGE('',*,*,#4962,.F.);
#6285=ORIENTED_EDGE('',*,*,#4960,.T.);
#6286=ORIENTED_EDGE('',*,*,#4963,.F.);
#6287=ORIENTED_EDGE('',*,*,#4957,.T.);
#6288=ORIENTED_EDGE('',*,*,#4953,.T.);
#6289=ORIENTED_EDGE('',*,*,#4964,.F.);
#6290=ORIENTED_EDGE('',*,*,#4965,.T.);
#6291=ORIENTED_EDGE('',*,*,#4966,.F.);
#6292=ORIENTED_EDGE('',*,*,#4967,.F.);
#6293=ORIENTED_EDGE('',*,*,#4968,.F.);
#6294=ORIENTED_EDGE('',*,*,#4969,.F.);
#6295=ORIENTED_EDGE('',*,*,#4970,.F.);
#6296=ORIENTED_EDGE('',*,*,#4965,.F.);
#6297=ORIENTED_EDGE('',*,*,#4971,.F.);
#6298=ORIENTED_EDGE('',*,*,#4967,.T.);
#6299=ORIENTED_EDGE('',*,*,#4972,.F.);
#6300=ORIENTED_EDGE('',*,*,#4973,.F.);
#6301=ORIENTED_EDGE('',*,*,#4971,.T.);
#6302=ORIENTED_EDGE('',*,*,#4974,.F.);
#6303=ORIENTED_EDGE('',*,*,#4968,.T.);
#6304=ORIENTED_EDGE('',*,*,#4964,.T.);
#6305=ORIENTED_EDGE('',*,*,#4975,.F.);
#6306=ORIENTED_EDGE('',*,*,#4976,.T.);
#6307=ORIENTED_EDGE('',*,*,#4977,.F.);
#6308=ORIENTED_EDGE('',*,*,#4978,.F.);
#6309=ORIENTED_EDGE('',*,*,#4979,.F.);
#6310=ORIENTED_EDGE('',*,*,#4980,.F.);
#6311=ORIENTED_EDGE('',*,*,#4981,.F.);
#6312=ORIENTED_EDGE('',*,*,#4976,.F.);
#6313=ORIENTED_EDGE('',*,*,#4982,.F.);
#6314=ORIENTED_EDGE('',*,*,#4978,.T.);
#6315=ORIENTED_EDGE('',*,*,#4983,.F.);
#6316=ORIENTED_EDGE('',*,*,#4984,.F.);
#6317=ORIENTED_EDGE('',*,*,#4982,.T.);
#6318=ORIENTED_EDGE('',*,*,#4985,.F.);
#6319=ORIENTED_EDGE('',*,*,#4979,.T.);
#6320=ORIENTED_EDGE('',*,*,#4975,.T.);
#6321=ORIENTED_EDGE('',*,*,#4986,.F.);
#6322=ORIENTED_EDGE('',*,*,#4987,.T.);
#6323=ORIENTED_EDGE('',*,*,#4988,.F.);
#6324=ORIENTED_EDGE('',*,*,#4989,.F.);
#6325=ORIENTED_EDGE('',*,*,#4990,.F.);
#6326=ORIENTED_EDGE('',*,*,#4991,.F.);
#6327=ORIENTED_EDGE('',*,*,#4992,.F.);
#6328=ORIENTED_EDGE('',*,*,#4987,.F.);
#6329=ORIENTED_EDGE('',*,*,#4993,.F.);
#6330=ORIENTED_EDGE('',*,*,#4989,.T.);
#6331=ORIENTED_EDGE('',*,*,#4994,.F.);
#6332=ORIENTED_EDGE('',*,*,#4995,.F.);
#6333=ORIENTED_EDGE('',*,*,#4993,.T.);
#6334=ORIENTED_EDGE('',*,*,#4996,.F.);
#6335=ORIENTED_EDGE('',*,*,#4990,.T.);
#6336=ORIENTED_EDGE('',*,*,#4986,.T.);
#6337=ORIENTED_EDGE('',*,*,#4997,.F.);
#6338=ORIENTED_EDGE('',*,*,#4998,.T.);
#6339=ORIENTED_EDGE('',*,*,#4999,.F.);
#6340=ORIENTED_EDGE('',*,*,#5000,.F.);
#6341=ORIENTED_EDGE('',*,*,#5001,.F.);
#6342=ORIENTED_EDGE('',*,*,#5002,.F.);
#6343=ORIENTED_EDGE('',*,*,#5003,.F.);
#6344=ORIENTED_EDGE('',*,*,#4998,.F.);
#6345=ORIENTED_EDGE('',*,*,#5004,.F.);
#6346=ORIENTED_EDGE('',*,*,#5000,.T.);
#6347=ORIENTED_EDGE('',*,*,#5005,.F.);
#6348=ORIENTED_EDGE('',*,*,#5006,.F.);
#6349=ORIENTED_EDGE('',*,*,#5004,.T.);
#6350=ORIENTED_EDGE('',*,*,#5007,.F.);
#6351=ORIENTED_EDGE('',*,*,#5001,.T.);
#6352=ORIENTED_EDGE('',*,*,#4997,.T.);
#6353=ORIENTED_EDGE('',*,*,#5008,.F.);
#6354=ORIENTED_EDGE('',*,*,#5009,.T.);
#6355=ORIENTED_EDGE('',*,*,#5010,.F.);
#6356=ORIENTED_EDGE('',*,*,#5011,.F.);
#6357=ORIENTED_EDGE('',*,*,#5012,.F.);
#6358=ORIENTED_EDGE('',*,*,#5013,.F.);
#6359=ORIENTED_EDGE('',*,*,#5014,.F.);
#6360=ORIENTED_EDGE('',*,*,#5009,.F.);
#6361=ORIENTED_EDGE('',*,*,#5015,.F.);
#6362=ORIENTED_EDGE('',*,*,#5011,.T.);
#6363=ORIENTED_EDGE('',*,*,#5016,.F.);
#6364=ORIENTED_EDGE('',*,*,#5017,.F.);
#6365=ORIENTED_EDGE('',*,*,#5015,.T.);
#6366=ORIENTED_EDGE('',*,*,#5018,.F.);
#6367=ORIENTED_EDGE('',*,*,#5012,.T.);
#6368=ORIENTED_EDGE('',*,*,#5008,.T.);
#6369=ORIENTED_EDGE('',*,*,#5019,.F.);
#6370=ORIENTED_EDGE('',*,*,#5020,.T.);
#6371=ORIENTED_EDGE('',*,*,#5021,.F.);
#6372=ORIENTED_EDGE('',*,*,#5022,.F.);
#6373=ORIENTED_EDGE('',*,*,#5023,.F.);
#6374=ORIENTED_EDGE('',*,*,#5024,.F.);
#6375=ORIENTED_EDGE('',*,*,#5025,.F.);
#6376=ORIENTED_EDGE('',*,*,#5020,.F.);
#6377=ORIENTED_EDGE('',*,*,#5026,.F.);
#6378=ORIENTED_EDGE('',*,*,#5022,.T.);
#6379=ORIENTED_EDGE('',*,*,#5027,.F.);
#6380=ORIENTED_EDGE('',*,*,#5028,.F.);
#6381=ORIENTED_EDGE('',*,*,#5026,.T.);
#6382=ORIENTED_EDGE('',*,*,#5029,.F.);
#6383=ORIENTED_EDGE('',*,*,#5023,.T.);
#6384=ORIENTED_EDGE('',*,*,#5019,.T.);
#6385=ORIENTED_EDGE('',*,*,#5030,.F.);
#6386=ORIENTED_EDGE('',*,*,#5031,.T.);
#6387=ORIENTED_EDGE('',*,*,#5032,.F.);
#6388=ORIENTED_EDGE('',*,*,#5033,.F.);
#6389=ORIENTED_EDGE('',*,*,#5034,.F.);
#6390=ORIENTED_EDGE('',*,*,#5035,.F.);
#6391=ORIENTED_EDGE('',*,*,#5036,.F.);
#6392=ORIENTED_EDGE('',*,*,#5031,.F.);
#6393=ORIENTED_EDGE('',*,*,#5037,.F.);
#6394=ORIENTED_EDGE('',*,*,#5033,.T.);
#6395=ORIENTED_EDGE('',*,*,#5038,.F.);
#6396=ORIENTED_EDGE('',*,*,#5039,.F.);
#6397=ORIENTED_EDGE('',*,*,#5037,.T.);
#6398=ORIENTED_EDGE('',*,*,#5040,.F.);
#6399=ORIENTED_EDGE('',*,*,#5034,.T.);
#6400=ORIENTED_EDGE('',*,*,#5030,.T.);
#6401=ORIENTED_EDGE('',*,*,#5041,.F.);
#6402=ORIENTED_EDGE('',*,*,#5042,.T.);
#6403=ORIENTED_EDGE('',*,*,#5043,.F.);
#6404=ORIENTED_EDGE('',*,*,#5044,.F.);
#6405=ORIENTED_EDGE('',*,*,#5045,.F.);
#6406=ORIENTED_EDGE('',*,*,#5046,.F.);
#6407=ORIENTED_EDGE('',*,*,#5047,.F.);
#6408=ORIENTED_EDGE('',*,*,#5042,.F.);
#6409=ORIENTED_EDGE('',*,*,#5048,.F.);
#6410=ORIENTED_EDGE('',*,*,#5044,.T.);
#6411=ORIENTED_EDGE('',*,*,#5049,.F.);
#6412=ORIENTED_EDGE('',*,*,#5050,.F.);
#6413=ORIENTED_EDGE('',*,*,#5048,.T.);
#6414=ORIENTED_EDGE('',*,*,#5051,.F.);
#6415=ORIENTED_EDGE('',*,*,#5045,.T.);
#6416=ORIENTED_EDGE('',*,*,#5041,.T.);
#6417=ORIENTED_EDGE('',*,*,#5052,.F.);
#6418=ORIENTED_EDGE('',*,*,#5053,.T.);
#6419=ORIENTED_EDGE('',*,*,#5054,.F.);
#6420=ORIENTED_EDGE('',*,*,#5055,.F.);
#6421=ORIENTED_EDGE('',*,*,#5056,.F.);
#6422=ORIENTED_EDGE('',*,*,#5057,.F.);
#6423=ORIENTED_EDGE('',*,*,#5058,.F.);
#6424=ORIENTED_EDGE('',*,*,#5053,.F.);
#6425=ORIENTED_EDGE('',*,*,#5059,.F.);
#6426=ORIENTED_EDGE('',*,*,#5055,.T.);
#6427=ORIENTED_EDGE('',*,*,#5060,.F.);
#6428=ORIENTED_EDGE('',*,*,#5061,.F.);
#6429=ORIENTED_EDGE('',*,*,#5059,.T.);
#6430=ORIENTED_EDGE('',*,*,#5062,.F.);
#6431=ORIENTED_EDGE('',*,*,#5056,.T.);
#6432=ORIENTED_EDGE('',*,*,#5052,.T.);
#6433=ORIENTED_EDGE('',*,*,#5063,.F.);
#6434=ORIENTED_EDGE('',*,*,#5064,.T.);
#6435=ORIENTED_EDGE('',*,*,#5065,.F.);
#6436=ORIENTED_EDGE('',*,*,#5066,.F.);
#6437=ORIENTED_EDGE('',*,*,#5067,.F.);
#6438=ORIENTED_EDGE('',*,*,#5068,.F.);
#6439=ORIENTED_EDGE('',*,*,#5069,.F.);
#6440=ORIENTED_EDGE('',*,*,#5064,.F.);
#6441=ORIENTED_EDGE('',*,*,#5070,.F.);
#6442=ORIENTED_EDGE('',*,*,#5066,.T.);
#6443=ORIENTED_EDGE('',*,*,#5071,.F.);
#6444=ORIENTED_EDGE('',*,*,#5072,.F.);
#6445=ORIENTED_EDGE('',*,*,#5070,.T.);
#6446=ORIENTED_EDGE('',*,*,#5073,.F.);
#6447=ORIENTED_EDGE('',*,*,#5067,.T.);
#6448=ORIENTED_EDGE('',*,*,#5063,.T.);
#6449=ORIENTED_EDGE('',*,*,#5074,.F.);
#6450=ORIENTED_EDGE('',*,*,#5075,.T.);
#6451=ORIENTED_EDGE('',*,*,#5076,.F.);
#6452=ORIENTED_EDGE('',*,*,#5077,.F.);
#6453=ORIENTED_EDGE('',*,*,#5078,.F.);
#6454=ORIENTED_EDGE('',*,*,#5079,.F.);
#6455=ORIENTED_EDGE('',*,*,#5080,.F.);
#6456=ORIENTED_EDGE('',*,*,#5075,.F.);
#6457=ORIENTED_EDGE('',*,*,#5081,.F.);
#6458=ORIENTED_EDGE('',*,*,#5077,.T.);
#6459=ORIENTED_EDGE('',*,*,#5082,.F.);
#6460=ORIENTED_EDGE('',*,*,#5083,.F.);
#6461=ORIENTED_EDGE('',*,*,#5081,.T.);
#6462=ORIENTED_EDGE('',*,*,#5084,.F.);
#6463=ORIENTED_EDGE('',*,*,#5078,.T.);
#6464=ORIENTED_EDGE('',*,*,#5074,.T.);
#6465=ORIENTED_EDGE('',*,*,#5085,.F.);
#6466=ORIENTED_EDGE('',*,*,#5086,.T.);
#6467=ORIENTED_EDGE('',*,*,#5087,.F.);
#6468=ORIENTED_EDGE('',*,*,#5088,.F.);
#6469=ORIENTED_EDGE('',*,*,#5089,.F.);
#6470=ORIENTED_EDGE('',*,*,#5090,.F.);
#6471=ORIENTED_EDGE('',*,*,#5091,.F.);
#6472=ORIENTED_EDGE('',*,*,#5086,.F.);
#6473=ORIENTED_EDGE('',*,*,#5092,.F.);
#6474=ORIENTED_EDGE('',*,*,#5088,.T.);
#6475=ORIENTED_EDGE('',*,*,#5093,.F.);
#6476=ORIENTED_EDGE('',*,*,#5094,.F.);
#6477=ORIENTED_EDGE('',*,*,#5092,.T.);
#6478=ORIENTED_EDGE('',*,*,#5095,.F.);
#6479=ORIENTED_EDGE('',*,*,#5089,.T.);
#6480=ORIENTED_EDGE('',*,*,#5085,.T.);
#6481=ORIENTED_EDGE('',*,*,#5096,.F.);
#6482=ORIENTED_EDGE('',*,*,#5097,.T.);
#6483=ORIENTED_EDGE('',*,*,#5098,.F.);
#6484=ORIENTED_EDGE('',*,*,#5099,.F.);
#6485=ORIENTED_EDGE('',*,*,#5100,.F.);
#6486=ORIENTED_EDGE('',*,*,#5101,.F.);
#6487=ORIENTED_EDGE('',*,*,#5102,.F.);
#6488=ORIENTED_EDGE('',*,*,#5097,.F.);
#6489=ORIENTED_EDGE('',*,*,#5103,.F.);
#6490=ORIENTED_EDGE('',*,*,#5099,.T.);
#6491=ORIENTED_EDGE('',*,*,#5104,.F.);
#6492=ORIENTED_EDGE('',*,*,#5105,.F.);
#6493=ORIENTED_EDGE('',*,*,#5103,.T.);
#6494=ORIENTED_EDGE('',*,*,#5106,.F.);
#6495=ORIENTED_EDGE('',*,*,#5100,.T.);
#6496=ORIENTED_EDGE('',*,*,#5096,.T.);
#6497=ORIENTED_EDGE('',*,*,#5107,.F.);
#6498=ORIENTED_EDGE('',*,*,#5108,.T.);
#6499=ORIENTED_EDGE('',*,*,#5109,.F.);
#6500=ORIENTED_EDGE('',*,*,#5110,.F.);
#6501=ORIENTED_EDGE('',*,*,#5111,.F.);
#6502=ORIENTED_EDGE('',*,*,#5112,.F.);
#6503=ORIENTED_EDGE('',*,*,#5113,.F.);
#6504=ORIENTED_EDGE('',*,*,#5108,.F.);
#6505=ORIENTED_EDGE('',*,*,#5114,.F.);
#6506=ORIENTED_EDGE('',*,*,#5110,.T.);
#6507=ORIENTED_EDGE('',*,*,#5115,.F.);
#6508=ORIENTED_EDGE('',*,*,#5116,.F.);
#6509=ORIENTED_EDGE('',*,*,#5114,.T.);
#6510=ORIENTED_EDGE('',*,*,#5117,.F.);
#6511=ORIENTED_EDGE('',*,*,#5111,.T.);
#6512=ORIENTED_EDGE('',*,*,#5107,.T.);
#6513=ORIENTED_EDGE('',*,*,#5118,.F.);
#6514=ORIENTED_EDGE('',*,*,#5119,.T.);
#6515=ORIENTED_EDGE('',*,*,#5120,.F.);
#6516=ORIENTED_EDGE('',*,*,#5121,.F.);
#6517=ORIENTED_EDGE('',*,*,#5122,.F.);
#6518=ORIENTED_EDGE('',*,*,#5123,.F.);
#6519=ORIENTED_EDGE('',*,*,#5124,.F.);
#6520=ORIENTED_EDGE('',*,*,#5119,.F.);
#6521=ORIENTED_EDGE('',*,*,#5125,.F.);
#6522=ORIENTED_EDGE('',*,*,#5121,.T.);
#6523=ORIENTED_EDGE('',*,*,#5126,.F.);
#6524=ORIENTED_EDGE('',*,*,#5127,.F.);
#6525=ORIENTED_EDGE('',*,*,#5125,.T.);
#6526=ORIENTED_EDGE('',*,*,#5128,.F.);
#6527=ORIENTED_EDGE('',*,*,#5122,.T.);
#6528=ORIENTED_EDGE('',*,*,#5118,.T.);
#6529=ORIENTED_EDGE('',*,*,#4818,.T.);
#6530=ORIENTED_EDGE('',*,*,#4812,.T.);
#6531=ORIENTED_EDGE('',*,*,#4816,.T.);
#6532=ORIENTED_EDGE('',*,*,#5129,.T.);
#6533=ORIENTED_EDGE('',*,*,#5126,.T.);
#6534=ORIENTED_EDGE('',*,*,#5120,.T.);
#6535=ORIENTED_EDGE('',*,*,#5124,.T.);
#6536=ORIENTED_EDGE('',*,*,#5130,.T.);
#6537=ORIENTED_EDGE('',*,*,#5131,.T.);
#6538=ORIENTED_EDGE('',*,*,#5132,.T.);
#6539=ORIENTED_EDGE('',*,*,#5133,.T.);
#6540=ORIENTED_EDGE('',*,*,#5134,.T.);
#6541=ORIENTED_EDGE('',*,*,#5049,.T.);
#6542=ORIENTED_EDGE('',*,*,#5043,.T.);
#6543=ORIENTED_EDGE('',*,*,#5047,.T.);
#6544=ORIENTED_EDGE('',*,*,#5135,.T.);
#6545=ORIENTED_EDGE('',*,*,#4972,.T.);
#6546=ORIENTED_EDGE('',*,*,#4966,.T.);
#6547=ORIENTED_EDGE('',*,*,#4970,.T.);
#6548=ORIENTED_EDGE('',*,*,#5136,.T.);
#6549=ORIENTED_EDGE('',*,*,#4961,.T.);
#6550=ORIENTED_EDGE('',*,*,#4955,.T.);
#6551=ORIENTED_EDGE('',*,*,#4959,.T.);
#6552=ORIENTED_EDGE('',*,*,#5137,.T.);
#6553=ORIENTED_EDGE('',*,*,#4983,.T.);
#6554=ORIENTED_EDGE('',*,*,#4977,.T.);
#6555=ORIENTED_EDGE('',*,*,#4981,.T.);
#6556=ORIENTED_EDGE('',*,*,#5138,.T.);
#6557=ORIENTED_EDGE('',*,*,#4950,.T.);
#6558=ORIENTED_EDGE('',*,*,#4944,.T.);
#6559=ORIENTED_EDGE('',*,*,#4948,.T.);
#6560=ORIENTED_EDGE('',*,*,#5139,.T.);
#6561=ORIENTED_EDGE('',*,*,#4994,.T.);
#6562=ORIENTED_EDGE('',*,*,#4988,.T.);
#6563=ORIENTED_EDGE('',*,*,#4992,.T.);
#6564=ORIENTED_EDGE('',*,*,#5140,.T.);
#6565=ORIENTED_EDGE('',*,*,#4939,.T.);
#6566=ORIENTED_EDGE('',*,*,#4933,.T.);
#6567=ORIENTED_EDGE('',*,*,#4937,.T.);
#6568=ORIENTED_EDGE('',*,*,#5141,.T.);
#6569=ORIENTED_EDGE('',*,*,#5005,.T.);
#6570=ORIENTED_EDGE('',*,*,#4999,.T.);
#6571=ORIENTED_EDGE('',*,*,#5003,.T.);
#6572=ORIENTED_EDGE('',*,*,#5142,.T.);
#6573=ORIENTED_EDGE('',*,*,#4928,.T.);
#6574=ORIENTED_EDGE('',*,*,#4922,.T.);
#6575=ORIENTED_EDGE('',*,*,#4926,.T.);
#6576=ORIENTED_EDGE('',*,*,#5143,.T.);
#6577=ORIENTED_EDGE('',*,*,#5016,.T.);
#6578=ORIENTED_EDGE('',*,*,#5010,.T.);
#6579=ORIENTED_EDGE('',*,*,#5014,.T.);
#6580=ORIENTED_EDGE('',*,*,#5144,.T.);
#6581=ORIENTED_EDGE('',*,*,#4917,.T.);
#6582=ORIENTED_EDGE('',*,*,#4911,.T.);
#6583=ORIENTED_EDGE('',*,*,#4915,.T.);
#6584=ORIENTED_EDGE('',*,*,#5145,.T.);
#6585=ORIENTED_EDGE('',*,*,#5027,.T.);
#6586=ORIENTED_EDGE('',*,*,#5021,.T.);
#6587=ORIENTED_EDGE('',*,*,#5025,.T.);
#6588=ORIENTED_EDGE('',*,*,#5146,.T.);
#6589=ORIENTED_EDGE('',*,*,#4906,.T.);
#6590=ORIENTED_EDGE('',*,*,#4900,.T.);
#6591=ORIENTED_EDGE('',*,*,#4904,.T.);
#6592=ORIENTED_EDGE('',*,*,#5147,.T.);
#6593=ORIENTED_EDGE('',*,*,#5038,.T.);
#6594=ORIENTED_EDGE('',*,*,#5032,.T.);
#6595=ORIENTED_EDGE('',*,*,#5036,.T.);
#6596=ORIENTED_EDGE('',*,*,#5148,.T.);
#6597=ORIENTED_EDGE('',*,*,#4895,.T.);
#6598=ORIENTED_EDGE('',*,*,#4889,.T.);
#6599=ORIENTED_EDGE('',*,*,#4893,.T.);
#6600=ORIENTED_EDGE('',*,*,#5149,.T.);
#6601=ORIENTED_EDGE('',*,*,#4884,.T.);
#6602=ORIENTED_EDGE('',*,*,#4878,.T.);
#6603=ORIENTED_EDGE('',*,*,#4882,.T.);
#6604=ORIENTED_EDGE('',*,*,#5150,.T.);
#6605=ORIENTED_EDGE('',*,*,#5060,.T.);
#6606=ORIENTED_EDGE('',*,*,#5054,.T.);
#6607=ORIENTED_EDGE('',*,*,#5058,.T.);
#6608=ORIENTED_EDGE('',*,*,#5151,.T.);
#6609=ORIENTED_EDGE('',*,*,#4873,.T.);
#6610=ORIENTED_EDGE('',*,*,#4867,.T.);
#6611=ORIENTED_EDGE('',*,*,#4871,.T.);
#6612=ORIENTED_EDGE('',*,*,#5152,.T.);
#6613=ORIENTED_EDGE('',*,*,#5071,.T.);
#6614=ORIENTED_EDGE('',*,*,#5065,.T.);
#6615=ORIENTED_EDGE('',*,*,#5069,.T.);
#6616=ORIENTED_EDGE('',*,*,#5153,.T.);
#6617=ORIENTED_EDGE('',*,*,#4862,.T.);
#6618=ORIENTED_EDGE('',*,*,#4856,.T.);
#6619=ORIENTED_EDGE('',*,*,#4860,.T.);
#6620=ORIENTED_EDGE('',*,*,#5154,.T.);
#6621=ORIENTED_EDGE('',*,*,#5082,.T.);
#6622=ORIENTED_EDGE('',*,*,#5076,.T.);
#6623=ORIENTED_EDGE('',*,*,#5080,.T.);
#6624=ORIENTED_EDGE('',*,*,#5155,.T.);
#6625=ORIENTED_EDGE('',*,*,#4851,.T.);
#6626=ORIENTED_EDGE('',*,*,#4845,.T.);
#6627=ORIENTED_EDGE('',*,*,#4849,.T.);
#6628=ORIENTED_EDGE('',*,*,#5156,.T.);
#6629=ORIENTED_EDGE('',*,*,#5093,.T.);
#6630=ORIENTED_EDGE('',*,*,#5087,.T.);
#6631=ORIENTED_EDGE('',*,*,#5091,.T.);
#6632=ORIENTED_EDGE('',*,*,#5157,.T.);
#6633=ORIENTED_EDGE('',*,*,#4840,.T.);
#6634=ORIENTED_EDGE('',*,*,#4834,.T.);
#6635=ORIENTED_EDGE('',*,*,#4838,.T.);
#6636=ORIENTED_EDGE('',*,*,#5158,.T.);
#6637=ORIENTED_EDGE('',*,*,#5104,.T.);
#6638=ORIENTED_EDGE('',*,*,#5098,.T.);
#6639=ORIENTED_EDGE('',*,*,#5102,.T.);
#6640=ORIENTED_EDGE('',*,*,#5159,.T.);
#6641=ORIENTED_EDGE('',*,*,#4829,.T.);
#6642=ORIENTED_EDGE('',*,*,#4823,.T.);
#6643=ORIENTED_EDGE('',*,*,#4827,.T.);
#6644=ORIENTED_EDGE('',*,*,#5160,.T.);
#6645=ORIENTED_EDGE('',*,*,#5115,.T.);
#6646=ORIENTED_EDGE('',*,*,#5109,.T.);
#6647=ORIENTED_EDGE('',*,*,#5113,.T.);
#6648=ORIENTED_EDGE('',*,*,#5161,.T.);
#6649=ORIENTED_EDGE('',*,*,#5162,.T.);
#6650=ORIENTED_EDGE('',*,*,#5163,.T.);
#6651=ORIENTED_EDGE('',*,*,#5164,.F.);
#6652=ORIENTED_EDGE('',*,*,#5165,.T.);
#6653=ORIENTED_EDGE('',*,*,#5163,.F.);
#6654=ORIENTED_EDGE('',*,*,#5165,.F.);
#6655=ORIENTED_EDGE('',*,*,#5166,.F.);
#6656=ORIENTED_EDGE('',*,*,#5167,.T.);
#6657=ORIENTED_EDGE('',*,*,#5162,.F.);
#6658=ORIENTED_EDGE('',*,*,#5167,.F.);
#6659=ORIENTED_EDGE('',*,*,#5168,.T.);
#6660=ORIENTED_EDGE('',*,*,#5169,.T.);
#6661=ORIENTED_EDGE('',*,*,#5132,.F.);
#6662=ORIENTED_EDGE('',*,*,#5170,.F.);
#6663=ORIENTED_EDGE('',*,*,#5171,.T.);
#6664=ORIENTED_EDGE('',*,*,#5170,.T.);
#6665=ORIENTED_EDGE('',*,*,#5131,.F.);
#6666=ORIENTED_EDGE('',*,*,#5172,.F.);
#6667=ORIENTED_EDGE('',*,*,#4819,.T.);
#6668=ORIENTED_EDGE('',*,*,#5161,.F.);
#6669=ORIENTED_EDGE('',*,*,#5112,.T.);
#6670=ORIENTED_EDGE('',*,*,#5117,.T.);
#6671=ORIENTED_EDGE('',*,*,#5116,.T.);
#6672=ORIENTED_EDGE('',*,*,#5160,.F.);
#6673=ORIENTED_EDGE('',*,*,#4826,.T.);
#6674=ORIENTED_EDGE('',*,*,#4831,.T.);
#6675=ORIENTED_EDGE('',*,*,#4830,.T.);
#6676=ORIENTED_EDGE('',*,*,#5159,.F.);
#6677=ORIENTED_EDGE('',*,*,#5101,.T.);
#6678=ORIENTED_EDGE('',*,*,#5106,.T.);
#6679=ORIENTED_EDGE('',*,*,#5105,.T.);
#6680=ORIENTED_EDGE('',*,*,#5158,.F.);
#6681=ORIENTED_EDGE('',*,*,#4837,.T.);
#6682=ORIENTED_EDGE('',*,*,#4842,.T.);
#6683=ORIENTED_EDGE('',*,*,#4841,.T.);
#6684=ORIENTED_EDGE('',*,*,#5157,.F.);
#6685=ORIENTED_EDGE('',*,*,#5090,.T.);
#6686=ORIENTED_EDGE('',*,*,#5095,.T.);
#6687=ORIENTED_EDGE('',*,*,#5094,.T.);
#6688=ORIENTED_EDGE('',*,*,#5156,.F.);
#6689=ORIENTED_EDGE('',*,*,#4848,.T.);
#6690=ORIENTED_EDGE('',*,*,#4853,.T.);
#6691=ORIENTED_EDGE('',*,*,#4852,.T.);
#6692=ORIENTED_EDGE('',*,*,#5155,.F.);
#6693=ORIENTED_EDGE('',*,*,#5079,.T.);
#6694=ORIENTED_EDGE('',*,*,#5084,.T.);
#6695=ORIENTED_EDGE('',*,*,#5083,.T.);
#6696=ORIENTED_EDGE('',*,*,#5154,.F.);
#6697=ORIENTED_EDGE('',*,*,#4859,.T.);
#6698=ORIENTED_EDGE('',*,*,#4864,.T.);
#6699=ORIENTED_EDGE('',*,*,#4863,.T.);
#6700=ORIENTED_EDGE('',*,*,#5153,.F.);
#6701=ORIENTED_EDGE('',*,*,#5068,.T.);
#6702=ORIENTED_EDGE('',*,*,#5073,.T.);
#6703=ORIENTED_EDGE('',*,*,#5072,.T.);
#6704=ORIENTED_EDGE('',*,*,#5152,.F.);
#6705=ORIENTED_EDGE('',*,*,#4870,.T.);
#6706=ORIENTED_EDGE('',*,*,#4875,.T.);
#6707=ORIENTED_EDGE('',*,*,#4874,.T.);
#6708=ORIENTED_EDGE('',*,*,#5151,.F.);
#6709=ORIENTED_EDGE('',*,*,#5057,.T.);
#6710=ORIENTED_EDGE('',*,*,#5062,.T.);
#6711=ORIENTED_EDGE('',*,*,#5061,.T.);
#6712=ORIENTED_EDGE('',*,*,#5150,.F.);
#6713=ORIENTED_EDGE('',*,*,#4881,.T.);
#6714=ORIENTED_EDGE('',*,*,#4886,.T.);
#6715=ORIENTED_EDGE('',*,*,#4885,.T.);
#6716=ORIENTED_EDGE('',*,*,#5149,.F.);
#6717=ORIENTED_EDGE('',*,*,#4892,.T.);
#6718=ORIENTED_EDGE('',*,*,#4897,.T.);
#6719=ORIENTED_EDGE('',*,*,#4896,.T.);
#6720=ORIENTED_EDGE('',*,*,#5148,.F.);
#6721=ORIENTED_EDGE('',*,*,#5035,.T.);
#6722=ORIENTED_EDGE('',*,*,#5040,.T.);
#6723=ORIENTED_EDGE('',*,*,#5039,.T.);
#6724=ORIENTED_EDGE('',*,*,#5147,.F.);
#6725=ORIENTED_EDGE('',*,*,#4903,.T.);
#6726=ORIENTED_EDGE('',*,*,#4908,.T.);
#6727=ORIENTED_EDGE('',*,*,#4907,.T.);
#6728=ORIENTED_EDGE('',*,*,#5146,.F.);
#6729=ORIENTED_EDGE('',*,*,#5024,.T.);
#6730=ORIENTED_EDGE('',*,*,#5029,.T.);
#6731=ORIENTED_EDGE('',*,*,#5028,.T.);
#6732=ORIENTED_EDGE('',*,*,#5145,.F.);
#6733=ORIENTED_EDGE('',*,*,#4914,.T.);
#6734=ORIENTED_EDGE('',*,*,#4919,.T.);
#6735=ORIENTED_EDGE('',*,*,#4918,.T.);
#6736=ORIENTED_EDGE('',*,*,#5144,.F.);
#6737=ORIENTED_EDGE('',*,*,#5013,.T.);
#6738=ORIENTED_EDGE('',*,*,#5018,.T.);
#6739=ORIENTED_EDGE('',*,*,#5017,.T.);
#6740=ORIENTED_EDGE('',*,*,#5143,.F.);
#6741=ORIENTED_EDGE('',*,*,#4925,.T.);
#6742=ORIENTED_EDGE('',*,*,#4930,.T.);
#6743=ORIENTED_EDGE('',*,*,#4929,.T.);
#6744=ORIENTED_EDGE('',*,*,#5142,.F.);
#6745=ORIENTED_EDGE('',*,*,#5002,.T.);
#6746=ORIENTED_EDGE('',*,*,#5007,.T.);
#6747=ORIENTED_EDGE('',*,*,#5006,.T.);
#6748=ORIENTED_EDGE('',*,*,#5141,.F.);
#6749=ORIENTED_EDGE('',*,*,#4936,.T.);
#6750=ORIENTED_EDGE('',*,*,#4941,.T.);
#6751=ORIENTED_EDGE('',*,*,#4940,.T.);
#6752=ORIENTED_EDGE('',*,*,#5140,.F.);
#6753=ORIENTED_EDGE('',*,*,#4991,.T.);
#6754=ORIENTED_EDGE('',*,*,#4996,.T.);
#6755=ORIENTED_EDGE('',*,*,#4995,.T.);
#6756=ORIENTED_EDGE('',*,*,#5139,.F.);
#6757=ORIENTED_EDGE('',*,*,#4947,.T.);
#6758=ORIENTED_EDGE('',*,*,#4952,.T.);
#6759=ORIENTED_EDGE('',*,*,#4951,.T.);
#6760=ORIENTED_EDGE('',*,*,#5138,.F.);
#6761=ORIENTED_EDGE('',*,*,#4980,.T.);
#6762=ORIENTED_EDGE('',*,*,#4985,.T.);
#6763=ORIENTED_EDGE('',*,*,#4984,.T.);
#6764=ORIENTED_EDGE('',*,*,#5137,.F.);
#6765=ORIENTED_EDGE('',*,*,#4958,.T.);
#6766=ORIENTED_EDGE('',*,*,#4963,.T.);
#6767=ORIENTED_EDGE('',*,*,#4962,.T.);
#6768=ORIENTED_EDGE('',*,*,#5136,.F.);
#6769=ORIENTED_EDGE('',*,*,#4969,.T.);
#6770=ORIENTED_EDGE('',*,*,#4974,.T.);
#6771=ORIENTED_EDGE('',*,*,#4973,.T.);
#6772=ORIENTED_EDGE('',*,*,#5135,.F.);
#6773=ORIENTED_EDGE('',*,*,#5046,.T.);
#6774=ORIENTED_EDGE('',*,*,#5051,.T.);
#6775=ORIENTED_EDGE('',*,*,#5050,.T.);
#6776=ORIENTED_EDGE('',*,*,#5134,.F.);
#6777=ORIENTED_EDGE('',*,*,#5173,.F.);
#6778=ORIENTED_EDGE('',*,*,#5174,.T.);
#6779=ORIENTED_EDGE('',*,*,#5172,.T.);
#6780=ORIENTED_EDGE('',*,*,#5130,.F.);
#6781=ORIENTED_EDGE('',*,*,#5123,.T.);
#6782=ORIENTED_EDGE('',*,*,#5128,.T.);
#6783=ORIENTED_EDGE('',*,*,#5127,.T.);
#6784=ORIENTED_EDGE('',*,*,#5129,.F.);
#6785=ORIENTED_EDGE('',*,*,#4815,.T.);
#6786=ORIENTED_EDGE('',*,*,#4820,.T.);
#6787=ORIENTED_EDGE('',*,*,#5175,.T.);
#6788=ORIENTED_EDGE('',*,*,#5173,.T.);
#6789=ORIENTED_EDGE('',*,*,#5133,.F.);
#6790=ORIENTED_EDGE('',*,*,#5169,.F.);
#6791=ORIENTED_EDGE('',*,*,#5175,.F.);
#6792=ORIENTED_EDGE('',*,*,#5168,.F.);
#6793=ORIENTED_EDGE('',*,*,#5171,.F.);
#6794=ORIENTED_EDGE('',*,*,#5174,.F.);
#6795=ORIENTED_EDGE('',*,*,#5164,.T.);
#6796=ORIENTED_EDGE('',*,*,#5166,.T.);
#8093=CYLINDRICAL_SURFACE('',#9146,0.225);
#8094=CYLINDRICAL_SURFACE('',#9148,0.225000000000001);
#8190=ADVANCED_FACE('',(#896),#502,.F.);
#8191=ADVANCED_FACE('',(#897),#503,.F.);
#8192=ADVANCED_FACE('',(#898),#504,.F.);
#8193=ADVANCED_FACE('',(#899),#505,.T.);
#8194=ADVANCED_FACE('',(#900),#506,.F.);
#8195=ADVANCED_FACE('',(#901),#507,.F.);
#8196=ADVANCED_FACE('',(#902),#508,.F.);
#8197=ADVANCED_FACE('',(#903),#509,.T.);
#8198=ADVANCED_FACE('',(#904),#510,.F.);
#8199=ADVANCED_FACE('',(#905),#511,.F.);
#8200=ADVANCED_FACE('',(#906),#512,.F.);
#8201=ADVANCED_FACE('',(#907),#513,.T.);
#8202=ADVANCED_FACE('',(#908),#514,.F.);
#8203=ADVANCED_FACE('',(#909),#515,.F.);
#8204=ADVANCED_FACE('',(#910),#516,.F.);
#8205=ADVANCED_FACE('',(#911),#517,.T.);
#8206=ADVANCED_FACE('',(#912),#518,.F.);
#8207=ADVANCED_FACE('',(#913),#519,.F.);
#8208=ADVANCED_FACE('',(#914),#520,.F.);
#8209=ADVANCED_FACE('',(#915),#521,.T.);
#8210=ADVANCED_FACE('',(#916),#522,.F.);
#8211=ADVANCED_FACE('',(#917),#523,.F.);
#8212=ADVANCED_FACE('',(#918),#524,.F.);
#8213=ADVANCED_FACE('',(#919),#525,.T.);
#8214=ADVANCED_FACE('',(#920),#526,.F.);
#8215=ADVANCED_FACE('',(#921),#527,.F.);
#8216=ADVANCED_FACE('',(#922),#528,.F.);
#8217=ADVANCED_FACE('',(#923),#529,.T.);
#8218=ADVANCED_FACE('',(#924),#530,.F.);
#8219=ADVANCED_FACE('',(#925),#531,.F.);
#8220=ADVANCED_FACE('',(#926),#532,.F.);
#8221=ADVANCED_FACE('',(#927),#533,.T.);
#8222=ADVANCED_FACE('',(#928),#534,.F.);
#8223=ADVANCED_FACE('',(#929),#535,.F.);
#8224=ADVANCED_FACE('',(#930),#536,.F.);
#8225=ADVANCED_FACE('',(#931),#537,.T.);
#8226=ADVANCED_FACE('',(#932),#538,.F.);
#8227=ADVANCED_FACE('',(#933),#539,.F.);
#8228=ADVANCED_FACE('',(#934),#540,.F.);
#8229=ADVANCED_FACE('',(#935),#541,.T.);
#8230=ADVANCED_FACE('',(#936),#542,.F.);
#8231=ADVANCED_FACE('',(#937),#543,.F.);
#8232=ADVANCED_FACE('',(#938),#544,.F.);
#8233=ADVANCED_FACE('',(#939),#545,.T.);
#8234=ADVANCED_FACE('',(#940),#546,.F.);
#8235=ADVANCED_FACE('',(#941),#547,.F.);
#8236=ADVANCED_FACE('',(#942),#548,.F.);
#8237=ADVANCED_FACE('',(#943),#549,.T.);
#8238=ADVANCED_FACE('',(#944),#550,.F.);
#8239=ADVANCED_FACE('',(#945),#551,.F.);
#8240=ADVANCED_FACE('',(#946),#552,.F.);
#8241=ADVANCED_FACE('',(#947),#553,.T.);
#8242=ADVANCED_FACE('',(#948),#554,.F.);
#8243=ADVANCED_FACE('',(#949),#555,.F.);
#8244=ADVANCED_FACE('',(#950),#556,.F.);
#8245=ADVANCED_FACE('',(#951),#557,.T.);
#8246=ADVANCED_FACE('',(#952),#558,.F.);
#8247=ADVANCED_FACE('',(#953),#559,.F.);
#8248=ADVANCED_FACE('',(#954),#560,.F.);
#8249=ADVANCED_FACE('',(#955),#561,.T.);
#8250=ADVANCED_FACE('',(#956),#562,.F.);
#8251=ADVANCED_FACE('',(#957),#563,.F.);
#8252=ADVANCED_FACE('',(#958),#564,.F.);
#8253=ADVANCED_FACE('',(#959),#565,.T.);
#8254=ADVANCED_FACE('',(#960),#566,.F.);
#8255=ADVANCED_FACE('',(#961),#567,.F.);
#8256=ADVANCED_FACE('',(#962),#568,.F.);
#8257=ADVANCED_FACE('',(#963),#569,.T.);
#8258=ADVANCED_FACE('',(#964),#570,.F.);
#8259=ADVANCED_FACE('',(#965),#571,.F.);
#8260=ADVANCED_FACE('',(#966),#572,.F.);
#8261=ADVANCED_FACE('',(#967),#573,.T.);
#8262=ADVANCED_FACE('',(#968),#574,.F.);
#8263=ADVANCED_FACE('',(#969),#575,.F.);
#8264=ADVANCED_FACE('',(#970),#576,.F.);
#8265=ADVANCED_FACE('',(#971),#577,.T.);
#8266=ADVANCED_FACE('',(#972),#578,.F.);
#8267=ADVANCED_FACE('',(#973),#579,.F.);
#8268=ADVANCED_FACE('',(#974),#580,.F.);
#8269=ADVANCED_FACE('',(#975),#581,.T.);
#8270=ADVANCED_FACE('',(#976),#582,.F.);
#8271=ADVANCED_FACE('',(#977),#583,.F.);
#8272=ADVANCED_FACE('',(#978),#584,.F.);
#8273=ADVANCED_FACE('',(#979),#585,.T.);
#8274=ADVANCED_FACE('',(#980),#586,.F.);
#8275=ADVANCED_FACE('',(#981),#587,.F.);
#8276=ADVANCED_FACE('',(#982),#588,.F.);
#8277=ADVANCED_FACE('',(#983),#589,.T.);
#8278=ADVANCED_FACE('',(#984),#590,.F.);
#8279=ADVANCED_FACE('',(#985),#591,.F.);
#8280=ADVANCED_FACE('',(#986),#592,.F.);
#8281=ADVANCED_FACE('',(#987),#593,.T.);
#8282=ADVANCED_FACE('',(#988),#594,.F.);
#8283=ADVANCED_FACE('',(#989),#595,.F.);
#8284=ADVANCED_FACE('',(#990),#596,.F.);
#8285=ADVANCED_FACE('',(#991),#597,.T.);
#8286=ADVANCED_FACE('',(#992),#598,.F.);
#8287=ADVANCED_FACE('',(#993),#599,.F.);
#8288=ADVANCED_FACE('',(#994),#600,.F.);
#8289=ADVANCED_FACE('',(#995),#601,.T.);
#8290=ADVANCED_FACE('',(#996),#602,.F.);
#8291=ADVANCED_FACE('',(#997),#603,.F.);
#8292=ADVANCED_FACE('',(#998),#604,.F.);
#8293=ADVANCED_FACE('',(#999),#605,.T.);
#8294=ADVANCED_FACE('',(#1000),#606,.F.);
#8295=ADVANCED_FACE('',(#1001),#607,.F.);
#8296=ADVANCED_FACE('',(#1002),#608,.F.);
#8297=ADVANCED_FACE('',(#1003),#609,.T.);
#8298=ADVANCED_FACE('',(#1004),#610,.F.);
#8299=ADVANCED_FACE('',(#1005),#611,.F.);
#8300=ADVANCED_FACE('',(#1006),#612,.F.);
#8301=ADVANCED_FACE('',(#1007),#613,.T.);
#8302=ADVANCED_FACE('',(#1008),#614,.F.);
#8303=ADVANCED_FACE('',(#1009),#615,.F.);
#8304=ADVANCED_FACE('',(#1010),#616,.F.);
#8305=ADVANCED_FACE('',(#1011),#617,.T.);
#8306=ADVANCED_FACE('',(#1012,#418,#419),#618,.T.);
#8307=ADVANCED_FACE('',(#1013),#8093,.F.);
#8308=ADVANCED_FACE('',(#1014),#8094,.F.);
#8309=ADVANCED_FACE('',(#1015),#619,.T.);
#8310=ADVANCED_FACE('',(#1016),#620,.T.);
#8311=ADVANCED_FACE('',(#1017),#621,.T.);
#8312=ADVANCED_FACE('',(#1018),#622,.T.);
#8313=ADVANCED_FACE('',(#1019,#420,#421),#623,.F.);
#8594=CLOSED_SHELL('',(#8190,#8191,#8192,#8193,#8194,#8195,#8196,#8197,
#8198,#8199,#8200,#8201,#8202,#8203,#8204,#8205,#8206,#8207,#8208,#8209,
#8210,#8211,#8212,#8213,#8214,#8215,#8216,#8217,#8218,#8219,#8220,#8221,
#8222,#8223,#8224,#8225,#8226,#8227,#8228,#8229,#8230,#8231,#8232,#8233,
#8234,#8235,#8236,#8237,#8238,#8239,#8240,#8241,#8242,#8243,#8244,#8245,
#8246,#8247,#8248,#8249,#8250,#8251,#8252,#8253,#8254,#8255,#8256,#8257,
#8258,#8259,#8260,#8261,#8262,#8263,#8264,#8265,#8266,#8267,#8268,#8269,
#8270,#8271,#8272,#8273,#8274,#8275,#8276,#8277,#8278,#8279,#8280,#8281,
#8282,#8283,#8284,#8285,#8286,#8287,#8288,#8289,#8290,#8291,#8292,#8293,
#8294,#8295,#8296,#8297,#8298,#8299,#8300,#8301,#8302,#8303,#8304,#8305,
#8306,#8307,#8308,#8309,#8310,#8311,#8312,#8313));
#9026=AXIS2_PLACEMENT_3D('',#12269,#9917,#9918);
#9027=AXIS2_PLACEMENT_3D('',#12270,#9919,#9920);
#9028=AXIS2_PLACEMENT_3D('',#12279,#9925,#9926);
#9029=AXIS2_PLACEMENT_3D('',#12285,#9930,#9931);
#9030=AXIS2_PLACEMENT_3D('',#12291,#9935,#9936);
#9031=AXIS2_PLACEMENT_3D('',#12293,#9938,#9939);
#9032=AXIS2_PLACEMENT_3D('',#12302,#9944,#9945);
#9033=AXIS2_PLACEMENT_3D('',#12308,#9949,#9950);
#9034=AXIS2_PLACEMENT_3D('',#12314,#9954,#9955);
#9035=AXIS2_PLACEMENT_3D('',#12316,#9957,#9958);
#9036=AXIS2_PLACEMENT_3D('',#12325,#9963,#9964);
#9037=AXIS2_PLACEMENT_3D('',#12331,#9968,#9969);
#9038=AXIS2_PLACEMENT_3D('',#12337,#9973,#9974);
#9039=AXIS2_PLACEMENT_3D('',#12339,#9976,#9977);
#9040=AXIS2_PLACEMENT_3D('',#12348,#9982,#9983);
#9041=AXIS2_PLACEMENT_3D('',#12354,#9987,#9988);
#9042=AXIS2_PLACEMENT_3D('',#12360,#9992,#9993);
#9043=AXIS2_PLACEMENT_3D('',#12362,#9995,#9996);
#9044=AXIS2_PLACEMENT_3D('',#12371,#10001,#10002);
#9045=AXIS2_PLACEMENT_3D('',#12377,#10006,#10007);
#9046=AXIS2_PLACEMENT_3D('',#12383,#10011,#10012);
#9047=AXIS2_PLACEMENT_3D('',#12385,#10014,#10015);
#9048=AXIS2_PLACEMENT_3D('',#12394,#10020,#10021);
#9049=AXIS2_PLACEMENT_3D('',#12400,#10025,#10026);
#9050=AXIS2_PLACEMENT_3D('',#12406,#10030,#10031);
#9051=AXIS2_PLACEMENT_3D('',#12408,#10033,#10034);
#9052=AXIS2_PLACEMENT_3D('',#12417,#10039,#10040);
#9053=AXIS2_PLACEMENT_3D('',#12423,#10044,#10045);
#9054=AXIS2_PLACEMENT_3D('',#12429,#10049,#10050);
#9055=AXIS2_PLACEMENT_3D('',#12431,#10052,#10053);
#9056=AXIS2_PLACEMENT_3D('',#12440,#10058,#10059);
#9057=AXIS2_PLACEMENT_3D('',#12446,#10063,#10064);
#9058=AXIS2_PLACEMENT_3D('',#12452,#10068,#10069);
#9059=AXIS2_PLACEMENT_3D('',#12454,#10071,#10072);
#9060=AXIS2_PLACEMENT_3D('',#12463,#10077,#10078);
#9061=AXIS2_PLACEMENT_3D('',#12469,#10082,#10083);
#9062=AXIS2_PLACEMENT_3D('',#12475,#10087,#10088);
#9063=AXIS2_PLACEMENT_3D('',#12477,#10090,#10091);
#9064=AXIS2_PLACEMENT_3D('',#12486,#10096,#10097);
#9065=AXIS2_PLACEMENT_3D('',#12492,#10101,#10102);
#9066=AXIS2_PLACEMENT_3D('',#12498,#10106,#10107);
#9067=AXIS2_PLACEMENT_3D('',#12500,#10109,#10110);
#9068=AXIS2_PLACEMENT_3D('',#12509,#10115,#10116);
#9069=AXIS2_PLACEMENT_3D('',#12515,#10120,#10121);
#9070=AXIS2_PLACEMENT_3D('',#12521,#10125,#10126);
#9071=AXIS2_PLACEMENT_3D('',#12523,#10128,#10129);
#9072=AXIS2_PLACEMENT_3D('',#12532,#10134,#10135);
#9073=AXIS2_PLACEMENT_3D('',#12538,#10139,#10140);
#9074=AXIS2_PLACEMENT_3D('',#12544,#10144,#10145);
#9075=AXIS2_PLACEMENT_3D('',#12546,#10147,#10148);
#9076=AXIS2_PLACEMENT_3D('',#12555,#10153,#10154);
#9077=AXIS2_PLACEMENT_3D('',#12561,#10158,#10159);
#9078=AXIS2_PLACEMENT_3D('',#12567,#10163,#10164);
#9079=AXIS2_PLACEMENT_3D('',#12569,#10166,#10167);
#9080=AXIS2_PLACEMENT_3D('',#12578,#10172,#10173);
#9081=AXIS2_PLACEMENT_3D('',#12584,#10177,#10178);
#9082=AXIS2_PLACEMENT_3D('',#12590,#10182,#10183);
#9083=AXIS2_PLACEMENT_3D('',#12592,#10185,#10186);
#9084=AXIS2_PLACEMENT_3D('',#12601,#10191,#10192);
#9085=AXIS2_PLACEMENT_3D('',#12607,#10196,#10197);
#9086=AXIS2_PLACEMENT_3D('',#12613,#10201,#10202);
#9087=AXIS2_PLACEMENT_3D('',#12615,#10204,#10205);
#9088=AXIS2_PLACEMENT_3D('',#12624,#10210,#10211);
#9089=AXIS2_PLACEMENT_3D('',#12630,#10215,#10216);
#9090=AXIS2_PLACEMENT_3D('',#12636,#10220,#10221);
#9091=AXIS2_PLACEMENT_3D('',#12638,#10223,#10224);
#9092=AXIS2_PLACEMENT_3D('',#12647,#10229,#10230);
#9093=AXIS2_PLACEMENT_3D('',#12653,#10234,#10235);
#9094=AXIS2_PLACEMENT_3D('',#12659,#10239,#10240);
#9095=AXIS2_PLACEMENT_3D('',#12661,#10242,#10243);
#9096=AXIS2_PLACEMENT_3D('',#12670,#10248,#10249);
#9097=AXIS2_PLACEMENT_3D('',#12676,#10253,#10254);
#9098=AXIS2_PLACEMENT_3D('',#12682,#10258,#10259);
#9099=AXIS2_PLACEMENT_3D('',#12684,#10261,#10262);
#9100=AXIS2_PLACEMENT_3D('',#12693,#10267,#10268);
#9101=AXIS2_PLACEMENT_3D('',#12699,#10272,#10273);
#9102=AXIS2_PLACEMENT_3D('',#12705,#10277,#10278);
#9103=AXIS2_PLACEMENT_3D('',#12707,#10280,#10281);
#9104=AXIS2_PLACEMENT_3D('',#12716,#10286,#10287);
#9105=AXIS2_PLACEMENT_3D('',#12722,#10291,#10292);
#9106=AXIS2_PLACEMENT_3D('',#12728,#10296,#10297);
#9107=AXIS2_PLACEMENT_3D('',#12730,#10299,#10300);
#9108=AXIS2_PLACEMENT_3D('',#12739,#10305,#10306);
#9109=AXIS2_PLACEMENT_3D('',#12745,#10310,#10311);
#9110=AXIS2_PLACEMENT_3D('',#12751,#10315,#10316);
#9111=AXIS2_PLACEMENT_3D('',#12753,#10318,#10319);
#9112=AXIS2_PLACEMENT_3D('',#12762,#10324,#10325);
#9113=AXIS2_PLACEMENT_3D('',#12768,#10329,#10330);
#9114=AXIS2_PLACEMENT_3D('',#12774,#10334,#10335);
#9115=AXIS2_PLACEMENT_3D('',#12776,#10337,#10338);
#9116=AXIS2_PLACEMENT_3D('',#12785,#10343,#10344);
#9117=AXIS2_PLACEMENT_3D('',#12791,#10348,#10349);
#9118=AXIS2_PLACEMENT_3D('',#12797,#10353,#10354);
#9119=AXIS2_PLACEMENT_3D('',#12799,#10356,#10357);
#9120=AXIS2_PLACEMENT_3D('',#12808,#10362,#10363);
#9121=AXIS2_PLACEMENT_3D('',#12814,#10367,#10368);
#9122=AXIS2_PLACEMENT_3D('',#12820,#10372,#10373);
#9123=AXIS2_PLACEMENT_3D('',#12822,#10375,#10376);
#9124=AXIS2_PLACEMENT_3D('',#12831,#10381,#10382);
#9125=AXIS2_PLACEMENT_3D('',#12837,#10386,#10387);
#9126=AXIS2_PLACEMENT_3D('',#12843,#10391,#10392);
#9127=AXIS2_PLACEMENT_3D('',#12845,#10394,#10395);
#9128=AXIS2_PLACEMENT_3D('',#12854,#10400,#10401);
#9129=AXIS2_PLACEMENT_3D('',#12860,#10405,#10406);
#9130=AXIS2_PLACEMENT_3D('',#12866,#10410,#10411);
#9131=AXIS2_PLACEMENT_3D('',#12868,#10413,#10414);
#9132=AXIS2_PLACEMENT_3D('',#12877,#10419,#10420);
#9133=AXIS2_PLACEMENT_3D('',#12883,#10424,#10425);
#9134=AXIS2_PLACEMENT_3D('',#12889,#10429,#10430);
#9135=AXIS2_PLACEMENT_3D('',#12891,#10432,#10433);
#9136=AXIS2_PLACEMENT_3D('',#12900,#10438,#10439);
#9137=AXIS2_PLACEMENT_3D('',#12906,#10443,#10444);
#9138=AXIS2_PLACEMENT_3D('',#12912,#10448,#10449);
#9139=AXIS2_PLACEMENT_3D('',#12914,#10451,#10452);
#9140=AXIS2_PLACEMENT_3D('',#12923,#10457,#10458);
#9141=AXIS2_PLACEMENT_3D('',#12929,#10462,#10463);
#9142=AXIS2_PLACEMENT_3D('',#12935,#10467,#10468);
#9143=AXIS2_PLACEMENT_3D('',#12937,#10470,#10471);
#9144=AXIS2_PLACEMENT_3D('',#12976,#10505,#10506);
#9145=AXIS2_PLACEMENT_3D('',#12978,#10507,#10508);
#9146=AXIS2_PLACEMENT_3D('',#12979,#10509,#10510);
#9147=AXIS2_PLACEMENT_3D('',#12981,#10511,#10512);
#9148=AXIS2_PLACEMENT_3D('',#12983,#10514,#10515);
#9149=AXIS2_PLACEMENT_3D('',#12985,#10516,#10517);
#9150=AXIS2_PLACEMENT_3D('',#12987,#10519,#10520);
#9151=AXIS2_PLACEMENT_3D('',#12993,#10524,#10525);
#9152=AXIS2_PLACEMENT_3D('',#12997,#10528,#10529);
#9153=AXIS2_PLACEMENT_3D('',#13001,#10532,#10533);
#9154=AXIS2_PLACEMENT_3D('',#13003,#10535,#10536);
#9917=DIRECTION('axis',(0.,0.,1.));
#9918=DIRECTION('refdir',(1.,0.,0.));
#9919=DIRECTION('center_axis',(0.,1.,0.));
#9920=DIRECTION('ref_axis',(-1.,0.,0.));
#9921=DIRECTION('',(-1.,0.,0.));
#9922=DIRECTION('',(0.,0.,1.));
#9923=DIRECTION('',(1.,0.,0.));
#9924=DIRECTION('',(0.,0.,1.));
#9925=DIRECTION('center_axis',(1.,0.,0.));
#9926=DIRECTION('ref_axis',(0.,1.,0.));
#9927=DIRECTION('',(0.,1.,0.));
#9928=DIRECTION('',(0.,0.,-1.));
#9929=DIRECTION('',(0.,-1.,0.));
#9930=DIRECTION('center_axis',(-1.,0.,0.));
#9931=DIRECTION('ref_axis',(0.,-1.,0.));
#9932=DIRECTION('',(0.,-1.,0.));
#9933=DIRECTION('',(0.,1.,0.));
#9934=DIRECTION('',(0.,0.,1.));
#9935=DIRECTION('center_axis',(0.,0.,1.));
#9936=DIRECTION('ref_axis',(1.,0.,0.));
#9937=DIRECTION('',(-1.,0.,0.));
#9938=DIRECTION('center_axis',(0.,1.,0.));
#9939=DIRECTION('ref_axis',(-1.,0.,0.));
#9940=DIRECTION('',(-1.,0.,0.));
#9941=DIRECTION('',(0.,0.,1.));
#9942=DIRECTION('',(1.,0.,0.));
#9943=DIRECTION('',(0.,0.,1.));
#9944=DIRECTION('center_axis',(1.,0.,0.));
#9945=DIRECTION('ref_axis',(0.,1.,0.));
#9946=DIRECTION('',(0.,1.,0.));
#9947=DIRECTION('',(0.,0.,-1.));
#9948=DIRECTION('',(0.,-1.,0.));
#9949=DIRECTION('center_axis',(-1.,0.,0.));
#9950=DIRECTION('ref_axis',(0.,-1.,0.));
#9951=DIRECTION('',(0.,-1.,0.));
#9952=DIRECTION('',(0.,1.,0.));
#9953=DIRECTION('',(0.,0.,1.));
#9954=DIRECTION('center_axis',(0.,0.,1.));
#9955=DIRECTION('ref_axis',(1.,0.,0.));
#9956=DIRECTION('',(-1.,0.,0.));
#9957=DIRECTION('center_axis',(0.,1.,0.));
#9958=DIRECTION('ref_axis',(-1.,0.,0.));
#9959=DIRECTION('',(-1.,0.,0.));
#9960=DIRECTION('',(0.,0.,1.));
#9961=DIRECTION('',(1.,0.,0.));
#9962=DIRECTION('',(0.,0.,1.));
#9963=DIRECTION('center_axis',(1.,0.,0.));
#9964=DIRECTION('ref_axis',(0.,1.,0.));
#9965=DIRECTION('',(0.,1.,0.));
#9966=DIRECTION('',(0.,0.,-1.));
#9967=DIRECTION('',(0.,-1.,0.));
#9968=DIRECTION('center_axis',(-1.,0.,0.));
#9969=DIRECTION('ref_axis',(0.,-1.,0.));
#9970=DIRECTION('',(0.,-1.,0.));
#9971=DIRECTION('',(0.,1.,0.));
#9972=DIRECTION('',(0.,0.,1.));
#9973=DIRECTION('center_axis',(0.,0.,1.));
#9974=DIRECTION('ref_axis',(1.,0.,0.));
#9975=DIRECTION('',(-1.,0.,0.));
#9976=DIRECTION('center_axis',(0.,1.,0.));
#9977=DIRECTION('ref_axis',(-1.,0.,0.));
#9978=DIRECTION('',(-1.,0.,0.));
#9979=DIRECTION('',(0.,0.,1.));
#9980=DIRECTION('',(1.,0.,0.));
#9981=DIRECTION('',(0.,0.,1.));
#9982=DIRECTION('center_axis',(1.,0.,0.));
#9983=DIRECTION('ref_axis',(0.,1.,0.));
#9984=DIRECTION('',(0.,1.,0.));
#9985=DIRECTION('',(0.,0.,-1.));
#9986=DIRECTION('',(0.,-1.,0.));
#9987=DIRECTION('center_axis',(-1.,0.,0.));
#9988=DIRECTION('ref_axis',(0.,-1.,0.));
#9989=DIRECTION('',(0.,-1.,0.));
#9990=DIRECTION('',(0.,1.,0.));
#9991=DIRECTION('',(0.,0.,1.));
#9992=DIRECTION('center_axis',(0.,0.,1.));
#9993=DIRECTION('ref_axis',(1.,0.,0.));
#9994=DIRECTION('',(-1.,0.,0.));
#9995=DIRECTION('center_axis',(0.,1.,0.));
#9996=DIRECTION('ref_axis',(-1.,0.,0.));
#9997=DIRECTION('',(-1.,0.,0.));
#9998=DIRECTION('',(0.,0.,1.));
#9999=DIRECTION('',(1.,0.,0.));
#10000=DIRECTION('',(0.,0.,1.));
#10001=DIRECTION('center_axis',(1.,0.,0.));
#10002=DIRECTION('ref_axis',(0.,1.,0.));
#10003=DIRECTION('',(0.,1.,0.));
#10004=DIRECTION('',(0.,0.,-1.));
#10005=DIRECTION('',(0.,-1.,0.));
#10006=DIRECTION('center_axis',(-1.,0.,0.));
#10007=DIRECTION('ref_axis',(0.,-1.,0.));
#10008=DIRECTION('',(0.,-1.,0.));
#10009=DIRECTION('',(0.,1.,0.));
#10010=DIRECTION('',(0.,0.,1.));
#10011=DIRECTION('center_axis',(0.,0.,1.));
#10012=DIRECTION('ref_axis',(1.,0.,0.));
#10013=DIRECTION('',(-1.,0.,0.));
#10014=DIRECTION('center_axis',(0.,1.,0.));
#10015=DIRECTION('ref_axis',(-1.,0.,0.));
#10016=DIRECTION('',(-1.,0.,0.));
#10017=DIRECTION('',(0.,0.,1.));
#10018=DIRECTION('',(1.,0.,0.));
#10019=DIRECTION('',(0.,0.,1.));
#10020=DIRECTION('center_axis',(1.,0.,0.));
#10021=DIRECTION('ref_axis',(0.,1.,0.));
#10022=DIRECTION('',(0.,1.,0.));
#10023=DIRECTION('',(0.,0.,-1.));
#10024=DIRECTION('',(0.,-1.,0.));
#10025=DIRECTION('center_axis',(-1.,0.,0.));
#10026=DIRECTION('ref_axis',(0.,-1.,0.));
#10027=DIRECTION('',(0.,-1.,0.));
#10028=DIRECTION('',(0.,1.,0.));
#10029=DIRECTION('',(0.,0.,1.));
#10030=DIRECTION('center_axis',(0.,0.,1.));
#10031=DIRECTION('ref_axis',(1.,0.,0.));
#10032=DIRECTION('',(-1.,0.,0.));
#10033=DIRECTION('center_axis',(0.,1.,0.));
#10034=DIRECTION('ref_axis',(-1.,0.,0.));
#10035=DIRECTION('',(-1.,0.,0.));
#10036=DIRECTION('',(0.,0.,1.));
#10037=DIRECTION('',(1.,0.,0.));
#10038=DIRECTION('',(0.,0.,1.));
#10039=DIRECTION('center_axis',(1.,0.,0.));
#10040=DIRECTION('ref_axis',(0.,1.,0.));
#10041=DIRECTION('',(0.,1.,0.));
#10042=DIRECTION('',(0.,0.,-1.));
#10043=DIRECTION('',(0.,-1.,0.));
#10044=DIRECTION('center_axis',(-1.,0.,0.));
#10045=DIRECTION('ref_axis',(0.,-1.,0.));
#10046=DIRECTION('',(0.,-1.,0.));
#10047=DIRECTION('',(0.,1.,0.));
#10048=DIRECTION('',(0.,0.,1.));
#10049=DIRECTION('center_axis',(0.,0.,1.));
#10050=DIRECTION('ref_axis',(1.,0.,0.));
#10051=DIRECTION('',(-1.,0.,0.));
#10052=DIRECTION('center_axis',(0.,1.,0.));
#10053=DIRECTION('ref_axis',(-1.,0.,0.));
#10054=DIRECTION('',(-1.,0.,0.));
#10055=DIRECTION('',(0.,0.,1.));
#10056=DIRECTION('',(1.,0.,0.));
#10057=DIRECTION('',(0.,0.,1.));
#10058=DIRECTION('center_axis',(1.,0.,0.));
#10059=DIRECTION('ref_axis',(0.,1.,0.));
#10060=DIRECTION('',(0.,1.,0.));
#10061=DIRECTION('',(0.,0.,-1.));
#10062=DIRECTION('',(0.,-1.,0.));
#10063=DIRECTION('center_axis',(-1.,0.,0.));
#10064=DIRECTION('ref_axis',(0.,-1.,0.));
#10065=DIRECTION('',(0.,-1.,0.));
#10066=DIRECTION('',(0.,1.,0.));
#10067=DIRECTION('',(0.,0.,1.));
#10068=DIRECTION('center_axis',(0.,0.,1.));
#10069=DIRECTION('ref_axis',(1.,0.,0.));
#10070=DIRECTION('',(-1.,0.,0.));
#10071=DIRECTION('center_axis',(0.,1.,0.));
#10072=DIRECTION('ref_axis',(-1.,0.,0.));
#10073=DIRECTION('',(-1.,0.,0.));
#10074=DIRECTION('',(0.,0.,1.));
#10075=DIRECTION('',(1.,0.,0.));
#10076=DIRECTION('',(0.,0.,1.));
#10077=DIRECTION('center_axis',(1.,0.,0.));
#10078=DIRECTION('ref_axis',(0.,1.,0.));
#10079=DIRECTION('',(0.,1.,0.));
#10080=DIRECTION('',(0.,0.,-1.));
#10081=DIRECTION('',(0.,-1.,0.));
#10082=DIRECTION('center_axis',(-1.,0.,0.));
#10083=DIRECTION('ref_axis',(0.,-1.,0.));
#10084=DIRECTION('',(0.,-1.,0.));
#10085=DIRECTION('',(0.,1.,0.));
#10086=DIRECTION('',(0.,0.,1.));
#10087=DIRECTION('center_axis',(0.,0.,1.));
#10088=DIRECTION('ref_axis',(1.,0.,0.));
#10089=DIRECTION('',(-1.,0.,0.));
#10090=DIRECTION('center_axis',(0.,1.,0.));
#10091=DIRECTION('ref_axis',(-1.,0.,0.));
#10092=DIRECTION('',(-1.,0.,0.));
#10093=DIRECTION('',(0.,0.,1.));
#10094=DIRECTION('',(1.,0.,0.));
#10095=DIRECTION('',(0.,0.,1.));
#10096=DIRECTION('center_axis',(1.,0.,0.));
#10097=DIRECTION('ref_axis',(0.,1.,0.));
#10098=DIRECTION('',(0.,1.,0.));
#10099=DIRECTION('',(0.,0.,-1.));
#10100=DIRECTION('',(0.,-1.,0.));
#10101=DIRECTION('center_axis',(-1.,0.,0.));
#10102=DIRECTION('ref_axis',(0.,-1.,0.));
#10103=DIRECTION('',(0.,-1.,0.));
#10104=DIRECTION('',(0.,1.,0.));
#10105=DIRECTION('',(0.,0.,1.));
#10106=DIRECTION('center_axis',(0.,0.,1.));
#10107=DIRECTION('ref_axis',(1.,0.,0.));
#10108=DIRECTION('',(-1.,0.,0.));
#10109=DIRECTION('center_axis',(0.,1.,0.));
#10110=DIRECTION('ref_axis',(-1.,0.,0.));
#10111=DIRECTION('',(-1.,0.,0.));
#10112=DIRECTION('',(0.,0.,1.));
#10113=DIRECTION('',(1.,0.,0.));
#10114=DIRECTION('',(0.,0.,1.));
#10115=DIRECTION('center_axis',(1.,0.,0.));
#10116=DIRECTION('ref_axis',(0.,1.,0.));
#10117=DIRECTION('',(0.,1.,0.));
#10118=DIRECTION('',(0.,0.,-1.));
#10119=DIRECTION('',(0.,-1.,0.));
#10120=DIRECTION('center_axis',(-1.,0.,0.));
#10121=DIRECTION('ref_axis',(0.,-1.,0.));
#10122=DIRECTION('',(0.,-1.,0.));
#10123=DIRECTION('',(0.,1.,0.));
#10124=DIRECTION('',(0.,0.,1.));
#10125=DIRECTION('center_axis',(0.,0.,1.));
#10126=DIRECTION('ref_axis',(1.,0.,0.));
#10127=DIRECTION('',(-1.,0.,0.));
#10128=DIRECTION('center_axis',(0.,1.,0.));
#10129=DIRECTION('ref_axis',(-1.,0.,0.));
#10130=DIRECTION('',(-1.,0.,0.));
#10131=DIRECTION('',(0.,0.,1.));
#10132=DIRECTION('',(1.,0.,0.));
#10133=DIRECTION('',(0.,0.,1.));
#10134=DIRECTION('center_axis',(1.,0.,0.));
#10135=DIRECTION('ref_axis',(0.,1.,0.));
#10136=DIRECTION('',(0.,1.,0.));
#10137=DIRECTION('',(0.,0.,-1.));
#10138=DIRECTION('',(0.,-1.,0.));
#10139=DIRECTION('center_axis',(-1.,0.,0.));
#10140=DIRECTION('ref_axis',(0.,-1.,0.));
#10141=DIRECTION('',(0.,-1.,0.));
#10142=DIRECTION('',(0.,1.,0.));
#10143=DIRECTION('',(0.,0.,1.));
#10144=DIRECTION('center_axis',(0.,0.,1.));
#10145=DIRECTION('ref_axis',(1.,0.,0.));
#10146=DIRECTION('',(-1.,0.,0.));
#10147=DIRECTION('center_axis',(0.,1.,0.));
#10148=DIRECTION('ref_axis',(-1.,0.,0.));
#10149=DIRECTION('',(-1.,0.,0.));
#10150=DIRECTION('',(0.,0.,1.));
#10151=DIRECTION('',(1.,0.,0.));
#10152=DIRECTION('',(0.,0.,1.));
#10153=DIRECTION('center_axis',(1.,0.,0.));
#10154=DIRECTION('ref_axis',(0.,1.,0.));
#10155=DIRECTION('',(0.,1.,0.));
#10156=DIRECTION('',(0.,0.,-1.));
#10157=DIRECTION('',(0.,-1.,0.));
#10158=DIRECTION('center_axis',(-1.,0.,0.));
#10159=DIRECTION('ref_axis',(0.,-1.,0.));
#10160=DIRECTION('',(0.,-1.,0.));
#10161=DIRECTION('',(0.,1.,0.));
#10162=DIRECTION('',(0.,0.,1.));
#10163=DIRECTION('center_axis',(0.,0.,1.));
#10164=DIRECTION('ref_axis',(1.,0.,0.));
#10165=DIRECTION('',(-1.,0.,0.));
#10166=DIRECTION('center_axis',(0.,1.,0.));
#10167=DIRECTION('ref_axis',(-1.,0.,0.));
#10168=DIRECTION('',(-1.,0.,0.));
#10169=DIRECTION('',(0.,0.,1.));
#10170=DIRECTION('',(1.,0.,0.));
#10171=DIRECTION('',(0.,0.,1.));
#10172=DIRECTION('center_axis',(1.,0.,0.));
#10173=DIRECTION('ref_axis',(0.,1.,0.));
#10174=DIRECTION('',(0.,1.,0.));
#10175=DIRECTION('',(0.,0.,-1.));
#10176=DIRECTION('',(0.,-1.,0.));
#10177=DIRECTION('center_axis',(-1.,0.,0.));
#10178=DIRECTION('ref_axis',(0.,-1.,0.));
#10179=DIRECTION('',(0.,-1.,0.));
#10180=DIRECTION('',(0.,1.,0.));
#10181=DIRECTION('',(0.,0.,1.));
#10182=DIRECTION('center_axis',(0.,0.,1.));
#10183=DIRECTION('ref_axis',(1.,0.,0.));
#10184=DIRECTION('',(-1.,0.,0.));
#10185=DIRECTION('center_axis',(0.,1.,0.));
#10186=DIRECTION('ref_axis',(-1.,0.,0.));
#10187=DIRECTION('',(-1.,0.,0.));
#10188=DIRECTION('',(0.,0.,1.));
#10189=DIRECTION('',(1.,0.,0.));
#10190=DIRECTION('',(0.,0.,1.));
#10191=DIRECTION('center_axis',(1.,0.,0.));
#10192=DIRECTION('ref_axis',(0.,1.,0.));
#10193=DIRECTION('',(0.,1.,0.));
#10194=DIRECTION('',(0.,0.,-1.));
#10195=DIRECTION('',(0.,-1.,0.));
#10196=DIRECTION('center_axis',(-1.,0.,0.));
#10197=DIRECTION('ref_axis',(0.,-1.,0.));
#10198=DIRECTION('',(0.,-1.,0.));
#10199=DIRECTION('',(0.,1.,0.));
#10200=DIRECTION('',(0.,0.,1.));
#10201=DIRECTION('center_axis',(0.,0.,1.));
#10202=DIRECTION('ref_axis',(1.,0.,0.));
#10203=DIRECTION('',(-1.,0.,0.));
#10204=DIRECTION('center_axis',(0.,1.,0.));
#10205=DIRECTION('ref_axis',(-1.,0.,0.));
#10206=DIRECTION('',(-1.,0.,0.));
#10207=DIRECTION('',(0.,0.,1.));
#10208=DIRECTION('',(1.,0.,0.));
#10209=DIRECTION('',(0.,0.,1.));
#10210=DIRECTION('center_axis',(1.,0.,0.));
#10211=DIRECTION('ref_axis',(0.,1.,0.));
#10212=DIRECTION('',(0.,1.,0.));
#10213=DIRECTION('',(0.,0.,-1.));
#10214=DIRECTION('',(0.,-1.,0.));
#10215=DIRECTION('center_axis',(-1.,0.,0.));
#10216=DIRECTION('ref_axis',(0.,-1.,0.));
#10217=DIRECTION('',(0.,-1.,0.));
#10218=DIRECTION('',(0.,1.,0.));
#10219=DIRECTION('',(0.,0.,1.));
#10220=DIRECTION('center_axis',(0.,0.,1.));
#10221=DIRECTION('ref_axis',(1.,0.,0.));
#10222=DIRECTION('',(-1.,0.,0.));
#10223=DIRECTION('center_axis',(0.,1.,0.));
#10224=DIRECTION('ref_axis',(-1.,0.,0.));
#10225=DIRECTION('',(-1.,0.,0.));
#10226=DIRECTION('',(0.,0.,1.));
#10227=DIRECTION('',(1.,0.,0.));
#10228=DIRECTION('',(0.,0.,1.));
#10229=DIRECTION('center_axis',(1.,0.,0.));
#10230=DIRECTION('ref_axis',(0.,1.,0.));
#10231=DIRECTION('',(0.,1.,0.));
#10232=DIRECTION('',(0.,0.,-1.));
#10233=DIRECTION('',(0.,-1.,0.));
#10234=DIRECTION('center_axis',(-1.,0.,0.));
#10235=DIRECTION('ref_axis',(0.,-1.,0.));
#10236=DIRECTION('',(0.,-1.,0.));
#10237=DIRECTION('',(0.,1.,0.));
#10238=DIRECTION('',(0.,0.,1.));
#10239=DIRECTION('center_axis',(0.,0.,1.));
#10240=DIRECTION('ref_axis',(1.,0.,0.));
#10241=DIRECTION('',(-1.,0.,0.));
#10242=DIRECTION('center_axis',(0.,1.,0.));
#10243=DIRECTION('ref_axis',(-1.,0.,0.));
#10244=DIRECTION('',(-1.,0.,0.));
#10245=DIRECTION('',(0.,0.,1.));
#10246=DIRECTION('',(1.,0.,0.));
#10247=DIRECTION('',(0.,0.,1.));
#10248=DIRECTION('center_axis',(1.,0.,0.));
#10249=DIRECTION('ref_axis',(0.,1.,0.));
#10250=DIRECTION('',(0.,1.,0.));
#10251=DIRECTION('',(0.,0.,-1.));
#10252=DIRECTION('',(0.,-1.,0.));
#10253=DIRECTION('center_axis',(-1.,0.,0.));
#10254=DIRECTION('ref_axis',(0.,-1.,0.));
#10255=DIRECTION('',(0.,-1.,0.));
#10256=DIRECTION('',(0.,1.,0.));
#10257=DIRECTION('',(0.,0.,1.));
#10258=DIRECTION('center_axis',(0.,0.,1.));
#10259=DIRECTION('ref_axis',(1.,0.,0.));
#10260=DIRECTION('',(-1.,0.,0.));
#10261=DIRECTION('center_axis',(0.,1.,0.));
#10262=DIRECTION('ref_axis',(-1.,0.,0.));
#10263=DIRECTION('',(-1.,0.,0.));
#10264=DIRECTION('',(0.,0.,1.));
#10265=DIRECTION('',(1.,0.,0.));
#10266=DIRECTION('',(0.,0.,1.));
#10267=DIRECTION('center_axis',(1.,0.,0.));
#10268=DIRECTION('ref_axis',(0.,1.,0.));
#10269=DIRECTION('',(0.,1.,0.));
#10270=DIRECTION('',(0.,0.,-1.));
#10271=DIRECTION('',(0.,-1.,0.));
#10272=DIRECTION('center_axis',(-1.,0.,0.));
#10273=DIRECTION('ref_axis',(0.,-1.,0.));
#10274=DIRECTION('',(0.,-1.,0.));
#10275=DIRECTION('',(0.,1.,0.));
#10276=DIRECTION('',(0.,0.,1.));
#10277=DIRECTION('center_axis',(0.,0.,1.));
#10278=DIRECTION('ref_axis',(1.,0.,0.));
#10279=DIRECTION('',(-1.,0.,0.));
#10280=DIRECTION('center_axis',(0.,1.,0.));
#10281=DIRECTION('ref_axis',(-1.,0.,0.));
#10282=DIRECTION('',(-1.,0.,0.));
#10283=DIRECTION('',(0.,0.,1.));
#10284=DIRECTION('',(1.,0.,0.));
#10285=DIRECTION('',(0.,0.,1.));
#10286=DIRECTION('center_axis',(1.,0.,0.));
#10287=DIRECTION('ref_axis',(0.,1.,0.));
#10288=DIRECTION('',(0.,1.,0.));
#10289=DIRECTION('',(0.,0.,-1.));
#10290=DIRECTION('',(0.,-1.,0.));
#10291=DIRECTION('center_axis',(-1.,0.,0.));
#10292=DIRECTION('ref_axis',(0.,-1.,0.));
#10293=DIRECTION('',(0.,-1.,0.));
#10294=DIRECTION('',(0.,1.,0.));
#10295=DIRECTION('',(0.,0.,1.));
#10296=DIRECTION('center_axis',(0.,0.,1.));
#10297=DIRECTION('ref_axis',(1.,0.,0.));
#10298=DIRECTION('',(-1.,0.,0.));
#10299=DIRECTION('center_axis',(0.,1.,0.));
#10300=DIRECTION('ref_axis',(-1.,0.,0.));
#10301=DIRECTION('',(-1.,0.,0.));
#10302=DIRECTION('',(0.,0.,1.));
#10303=DIRECTION('',(1.,0.,0.));
#10304=DIRECTION('',(0.,0.,1.));
#10305=DIRECTION('center_axis',(1.,0.,0.));
#10306=DIRECTION('ref_axis',(0.,1.,0.));
#10307=DIRECTION('',(0.,1.,0.));
#10308=DIRECTION('',(0.,0.,-1.));
#10309=DIRECTION('',(0.,-1.,0.));
#10310=DIRECTION('center_axis',(-1.,0.,0.));
#10311=DIRECTION('ref_axis',(0.,-1.,0.));
#10312=DIRECTION('',(0.,-1.,0.));
#10313=DIRECTION('',(0.,1.,0.));
#10314=DIRECTION('',(0.,0.,1.));
#10315=DIRECTION('center_axis',(0.,0.,1.));
#10316=DIRECTION('ref_axis',(1.,0.,0.));
#10317=DIRECTION('',(-1.,0.,0.));
#10318=DIRECTION('center_axis',(0.,1.,0.));
#10319=DIRECTION('ref_axis',(-1.,0.,0.));
#10320=DIRECTION('',(-1.,0.,0.));
#10321=DIRECTION('',(0.,0.,1.));
#10322=DIRECTION('',(1.,0.,0.));
#10323=DIRECTION('',(0.,0.,1.));
#10324=DIRECTION('center_axis',(1.,0.,0.));
#10325=DIRECTION('ref_axis',(0.,1.,0.));
#10326=DIRECTION('',(0.,1.,0.));
#10327=DIRECTION('',(0.,0.,-1.));
#10328=DIRECTION('',(0.,-1.,0.));
#10329=DIRECTION('center_axis',(-1.,0.,0.));
#10330=DIRECTION('ref_axis',(0.,-1.,0.));
#10331=DIRECTION('',(0.,-1.,0.));
#10332=DIRECTION('',(0.,1.,0.));
#10333=DIRECTION('',(0.,0.,1.));
#10334=DIRECTION('center_axis',(0.,0.,1.));
#10335=DIRECTION('ref_axis',(1.,0.,0.));
#10336=DIRECTION('',(-1.,0.,0.));
#10337=DIRECTION('center_axis',(0.,1.,0.));
#10338=DIRECTION('ref_axis',(-1.,0.,0.));
#10339=DIRECTION('',(-1.,0.,0.));
#10340=DIRECTION('',(0.,0.,1.));
#10341=DIRECTION('',(1.,0.,0.));
#10342=DIRECTION('',(0.,0.,1.));
#10343=DIRECTION('center_axis',(1.,0.,0.));
#10344=DIRECTION('ref_axis',(0.,1.,0.));
#10345=DIRECTION('',(0.,1.,0.));
#10346=DIRECTION('',(0.,0.,-1.));
#10347=DIRECTION('',(0.,-1.,0.));
#10348=DIRECTION('center_axis',(-1.,0.,0.));
#10349=DIRECTION('ref_axis',(0.,-1.,0.));
#10350=DIRECTION('',(0.,-1.,0.));
#10351=DIRECTION('',(0.,1.,0.));
#10352=DIRECTION('',(0.,0.,1.));
#10353=DIRECTION('center_axis',(0.,0.,1.));
#10354=DIRECTION('ref_axis',(1.,0.,0.));
#10355=DIRECTION('',(-1.,0.,0.));
#10356=DIRECTION('center_axis',(0.,1.,0.));
#10357=DIRECTION('ref_axis',(-1.,0.,0.));
#10358=DIRECTION('',(-1.,0.,0.));
#10359=DIRECTION('',(0.,0.,1.));
#10360=DIRECTION('',(1.,0.,0.));
#10361=DIRECTION('',(0.,0.,1.));
#10362=DIRECTION('center_axis',(1.,0.,0.));
#10363=DIRECTION('ref_axis',(0.,1.,0.));
#10364=DIRECTION('',(0.,1.,0.));
#10365=DIRECTION('',(0.,0.,-1.));
#10366=DIRECTION('',(0.,-1.,0.));
#10367=DIRECTION('center_axis',(-1.,0.,0.));
#10368=DIRECTION('ref_axis',(0.,-1.,0.));
#10369=DIRECTION('',(0.,-1.,0.));
#10370=DIRECTION('',(0.,1.,0.));
#10371=DIRECTION('',(0.,0.,1.));
#10372=DIRECTION('center_axis',(0.,0.,1.));
#10373=DIRECTION('ref_axis',(1.,0.,0.));
#10374=DIRECTION('',(-1.,0.,0.));
#10375=DIRECTION('center_axis',(0.,1.,0.));
#10376=DIRECTION('ref_axis',(-1.,0.,0.));
#10377=DIRECTION('',(-1.,0.,0.));
#10378=DIRECTION('',(0.,0.,1.));
#10379=DIRECTION('',(1.,0.,0.));
#10380=DIRECTION('',(0.,0.,1.));
#10381=DIRECTION('center_axis',(1.,0.,0.));
#10382=DIRECTION('ref_axis',(0.,1.,0.));
#10383=DIRECTION('',(0.,1.,0.));
#10384=DIRECTION('',(0.,0.,-1.));
#10385=DIRECTION('',(0.,-1.,0.));
#10386=DIRECTION('center_axis',(-1.,0.,0.));
#10387=DIRECTION('ref_axis',(0.,-1.,0.));
#10388=DIRECTION('',(0.,-1.,0.));
#10389=DIRECTION('',(0.,1.,0.));
#10390=DIRECTION('',(0.,0.,1.));
#10391=DIRECTION('center_axis',(0.,0.,1.));
#10392=DIRECTION('ref_axis',(1.,0.,0.));
#10393=DIRECTION('',(-1.,0.,0.));
#10394=DIRECTION('center_axis',(0.,1.,0.));
#10395=DIRECTION('ref_axis',(-1.,0.,0.));
#10396=DIRECTION('',(-1.,0.,0.));
#10397=DIRECTION('',(0.,0.,1.));
#10398=DIRECTION('',(1.,0.,0.));
#10399=DIRECTION('',(0.,0.,1.));
#10400=DIRECTION('center_axis',(1.,0.,0.));
#10401=DIRECTION('ref_axis',(0.,1.,0.));
#10402=DIRECTION('',(0.,1.,0.));
#10403=DIRECTION('',(0.,0.,-1.));
#10404=DIRECTION('',(0.,-1.,0.));
#10405=DIRECTION('center_axis',(-1.,0.,0.));
#10406=DIRECTION('ref_axis',(0.,-1.,0.));
#10407=DIRECTION('',(0.,-1.,0.));
#10408=DIRECTION('',(0.,1.,0.));
#10409=DIRECTION('',(0.,0.,1.));
#10410=DIRECTION('center_axis',(0.,0.,1.));
#10411=DIRECTION('ref_axis',(1.,0.,0.));
#10412=DIRECTION('',(-1.,0.,0.));
#10413=DIRECTION('center_axis',(0.,1.,0.));
#10414=DIRECTION('ref_axis',(-1.,0.,0.));
#10415=DIRECTION('',(-1.,0.,0.));
#10416=DIRECTION('',(0.,0.,1.));
#10417=DIRECTION('',(1.,0.,0.));
#10418=DIRECTION('',(0.,0.,1.));
#10419=DIRECTION('center_axis',(1.,0.,0.));
#10420=DIRECTION('ref_axis',(0.,1.,0.));
#10421=DIRECTION('',(0.,1.,0.));
#10422=DIRECTION('',(0.,0.,-1.));
#10423=DIRECTION('',(0.,-1.,0.));
#10424=DIRECTION('center_axis',(-1.,0.,0.));
#10425=DIRECTION('ref_axis',(0.,-1.,0.));
#10426=DIRECTION('',(0.,-1.,0.));
#10427=DIRECTION('',(0.,1.,0.));
#10428=DIRECTION('',(0.,0.,1.));
#10429=DIRECTION('center_axis',(0.,0.,1.));
#10430=DIRECTION('ref_axis',(1.,0.,0.));
#10431=DIRECTION('',(-1.,0.,0.));
#10432=DIRECTION('center_axis',(0.,1.,0.));
#10433=DIRECTION('ref_axis',(-1.,0.,0.));
#10434=DIRECTION('',(-1.,0.,0.));
#10435=DIRECTION('',(0.,0.,1.));
#10436=DIRECTION('',(1.,0.,0.));
#10437=DIRECTION('',(0.,0.,1.));
#10438=DIRECTION('center_axis',(1.,0.,0.));
#10439=DIRECTION('ref_axis',(0.,1.,0.));
#10440=DIRECTION('',(0.,1.,0.));
#10441=DIRECTION('',(0.,0.,-1.));
#10442=DIRECTION('',(0.,-1.,0.));
#10443=DIRECTION('center_axis',(-1.,0.,0.));
#10444=DIRECTION('ref_axis',(0.,-1.,0.));
#10445=DIRECTION('',(0.,-1.,0.));
#10446=DIRECTION('',(0.,1.,0.));
#10447=DIRECTION('',(0.,0.,1.));
#10448=DIRECTION('center_axis',(0.,0.,1.));
#10449=DIRECTION('ref_axis',(1.,0.,0.));
#10450=DIRECTION('',(-1.,0.,0.));
#10451=DIRECTION('center_axis',(0.,1.,0.));
#10452=DIRECTION('ref_axis',(-1.,0.,0.));
#10453=DIRECTION('',(-1.,0.,0.));
#10454=DIRECTION('',(0.,0.,1.));
#10455=DIRECTION('',(1.,0.,0.));
#10456=DIRECTION('',(0.,0.,1.));
#10457=DIRECTION('center_axis',(1.,0.,0.));
#10458=DIRECTION('ref_axis',(0.,1.,0.));
#10459=DIRECTION('',(0.,1.,0.));
#10460=DIRECTION('',(0.,0.,-1.));
#10461=DIRECTION('',(0.,-1.,0.));
#10462=DIRECTION('center_axis',(-1.,0.,0.));
#10463=DIRECTION('ref_axis',(0.,-1.,0.));
#10464=DIRECTION('',(0.,-1.,0.));
#10465=DIRECTION('',(0.,1.,0.));
#10466=DIRECTION('',(0.,0.,1.));
#10467=DIRECTION('center_axis',(0.,0.,1.));
#10468=DIRECTION('ref_axis',(1.,0.,0.));
#10469=DIRECTION('',(-1.,0.,0.));
#10470=DIRECTION('center_axis',(0.,0.,1.));
#10471=DIRECTION('ref_axis',(1.,0.,0.));
#10472=DIRECTION('',(1.,0.,0.));
#10473=DIRECTION('',(1.,0.,0.));
#10474=DIRECTION('',(0.,1.,0.));
#10475=DIRECTION('',(-1.,0.,0.));
#10476=DIRECTION('',(0.,-1.,0.));
#10477=DIRECTION('',(1.,0.,0.));
#10478=DIRECTION('',(1.,0.,0.));
#10479=DIRECTION('',(1.,0.,0.));
#10480=DIRECTION('',(1.,0.,0.));
#10481=DIRECTION('',(1.,0.,0.));
#10482=DIRECTION('',(1.,0.,0.));
#10483=DIRECTION('',(1.,0.,0.));
#10484=DIRECTION('',(1.,0.,0.));
#10485=DIRECTION('',(1.,0.,0.));
#10486=DIRECTION('',(1.,0.,0.));
#10487=DIRECTION('',(1.,0.,0.));
#10488=DIRECTION('',(1.,0.,0.));
#10489=DIRECTION('',(1.,0.,0.));
#10490=DIRECTION('',(1.,0.,0.));
#10491=DIRECTION('',(1.,0.,0.));
#10492=DIRECTION('',(1.,0.,0.));
#10493=DIRECTION('',(1.,0.,0.));
#10494=DIRECTION('',(1.,0.,0.));
#10495=DIRECTION('',(1.,0.,0.));
#10496=DIRECTION('',(1.,0.,0.));
#10497=DIRECTION('',(1.,0.,0.));
#10498=DIRECTION('',(1.,0.,0.));
#10499=DIRECTION('',(1.,0.,0.));
#10500=DIRECTION('',(1.,0.,0.));
#10501=DIRECTION('',(1.,0.,0.));
#10502=DIRECTION('',(1.,0.,0.));
#10503=DIRECTION('',(1.,0.,0.));
#10504=DIRECTION('',(1.,0.,0.));
#10505=DIRECTION('center_axis',(0.,0.,-1.));
#10506=DIRECTION('ref_axis',(1.,0.,0.));
#10507=DIRECTION('center_axis',(0.,0.,-1.));
#10508=DIRECTION('ref_axis',(1.,0.,0.));
#10509=DIRECTION('center_axis',(0.,0.,1.));
#10510=DIRECTION('ref_axis',(1.,0.,0.));
#10511=DIRECTION('center_axis',(0.,0.,1.));
#10512=DIRECTION('ref_axis',(1.,0.,0.));
#10513=DIRECTION('',(0.,0.,1.));
#10514=DIRECTION('center_axis',(0.,0.,1.));
#10515=DIRECTION('ref_axis',(1.,0.,0.));
#10516=DIRECTION('center_axis',(0.,0.,1.));
#10517=DIRECTION('ref_axis',(1.,0.,0.));
#10518=DIRECTION('',(0.,0.,1.));
#10519=DIRECTION('center_axis',(0.,1.,0.));
#10520=DIRECTION('ref_axis',(-1.,0.,0.));
#10521=DIRECTION('',(-1.,0.,0.));
#10522=DIRECTION('',(0.,0.,1.));
#10523=DIRECTION('',(0.,0.,1.));
#10524=DIRECTION('center_axis',(1.,0.,0.));
#10525=DIRECTION('ref_axis',(0.,1.,0.));
#10526=DIRECTION('',(0.,1.,0.));
#10527=DIRECTION('',(0.,0.,1.));
#10528=DIRECTION('center_axis',(0.,-1.,0.));
#10529=DIRECTION('ref_axis',(1.,0.,0.));
#10530=DIRECTION('',(0.,0.,1.));
#10531=DIRECTION('',(1.,0.,0.));
#10532=DIRECTION('center_axis',(-1.,0.,0.));
#10533=DIRECTION('ref_axis',(0.,-1.,0.));
#10534=DIRECTION('',(0.,-1.,0.));
#10535=DIRECTION('center_axis',(0.,0.,1.));
#10536=DIRECTION('ref_axis',(1.,0.,0.));
#12269=CARTESIAN_POINT('',(0.,0.,0.));
#12270=CARTESIAN_POINT('Origin',(17.51,4.3,2.98));
#12271=CARTESIAN_POINT('',(17.51,4.3,2.98));
#12272=CARTESIAN_POINT('',(17.49,4.3,2.98));
#12273=CARTESIAN_POINT('',(17.51,4.3,2.98));
#12274=CARTESIAN_POINT('',(17.51,4.3,3.));
#12275=CARTESIAN_POINT('',(17.51,4.3,2.98));
#12276=CARTESIAN_POINT('',(17.49,4.3,3.));
#12277=CARTESIAN_POINT('',(14.255,4.3,3.));
#12278=CARTESIAN_POINT('',(17.49,4.3,2.98));
#12279=CARTESIAN_POINT('Origin',(17.51,4.,2.98));
#12280=CARTESIAN_POINT('',(17.51,4.,2.98));
#12281=CARTESIAN_POINT('',(17.51,4.,2.98));
#12282=CARTESIAN_POINT('',(17.51,4.,3.));
#12283=CARTESIAN_POINT('',(17.51,4.,2.89));
#12284=CARTESIAN_POINT('',(17.51,4.2,3.));
#12285=CARTESIAN_POINT('Origin',(17.49,4.3,2.98));
#12286=CARTESIAN_POINT('',(17.49,4.,2.98));
#12287=CARTESIAN_POINT('',(17.49,4.3,2.98));
#12288=CARTESIAN_POINT('',(17.49,4.,3.));
#12289=CARTESIAN_POINT('',(17.49,4.35,3.));
#12290=CARTESIAN_POINT('',(17.49,4.,2.89));
#12291=CARTESIAN_POINT('Origin',(17.5,4.15,2.98));
#12292=CARTESIAN_POINT('',(9.25,4.,2.98));
#12293=CARTESIAN_POINT('Origin',(16.51,4.3,2.98));
#12294=CARTESIAN_POINT('',(16.51,4.3,2.98));
#12295=CARTESIAN_POINT('',(16.49,4.3,2.98));
#12296=CARTESIAN_POINT('',(16.51,4.3,2.98));
#12297=CARTESIAN_POINT('',(16.51,4.3,3.));
#12298=CARTESIAN_POINT('',(16.51,4.3,2.98));
#12299=CARTESIAN_POINT('',(16.49,4.3,3.));
#12300=CARTESIAN_POINT('',(13.755,4.3,3.));
#12301=CARTESIAN_POINT('',(16.49,4.3,2.98));
#12302=CARTESIAN_POINT('Origin',(16.51,4.,2.98));
#12303=CARTESIAN_POINT('',(16.51,4.,2.98));
#12304=CARTESIAN_POINT('',(16.51,4.,2.98));
#12305=CARTESIAN_POINT('',(16.51,4.,3.));
#12306=CARTESIAN_POINT('',(16.51,4.,2.89));
#12307=CARTESIAN_POINT('',(16.51,4.2,3.));
#12308=CARTESIAN_POINT('Origin',(16.49,4.3,2.98));
#12309=CARTESIAN_POINT('',(16.49,4.,2.98));
#12310=CARTESIAN_POINT('',(16.49,4.3,2.98));
#12311=CARTESIAN_POINT('',(16.49,4.,3.));
#12312=CARTESIAN_POINT('',(16.49,4.35,3.));
#12313=CARTESIAN_POINT('',(16.49,4.,2.89));
#12314=CARTESIAN_POINT('Origin',(16.5,4.15,2.98));
#12315=CARTESIAN_POINT('',(8.75,4.,2.98));
#12316=CARTESIAN_POINT('Origin',(15.51,4.3,2.98));
#12317=CARTESIAN_POINT('',(15.51,4.3,2.98));
#12318=CARTESIAN_POINT('',(15.49,4.3,2.98));
#12319=CARTESIAN_POINT('',(15.51,4.3,2.98));
#12320=CARTESIAN_POINT('',(15.51,4.3,3.));
#12321=CARTESIAN_POINT('',(15.51,4.3,2.98));
#12322=CARTESIAN_POINT('',(15.49,4.3,3.));
#12323=CARTESIAN_POINT('',(13.255,4.3,3.));
#12324=CARTESIAN_POINT('',(15.49,4.3,2.98));
#12325=CARTESIAN_POINT('Origin',(15.51,4.,2.98));
#12326=CARTESIAN_POINT('',(15.51,4.,2.98));
#12327=CARTESIAN_POINT('',(15.51,4.,2.98));
#12328=CARTESIAN_POINT('',(15.51,4.,3.));
#12329=CARTESIAN_POINT('',(15.51,4.,2.89));
#12330=CARTESIAN_POINT('',(15.51,4.2,3.));
#12331=CARTESIAN_POINT('Origin',(15.49,4.3,2.98));
#12332=CARTESIAN_POINT('',(15.49,4.,2.98));
#12333=CARTESIAN_POINT('',(15.49,4.3,2.98));
#12334=CARTESIAN_POINT('',(15.49,4.,3.));
#12335=CARTESIAN_POINT('',(15.49,4.35,3.));
#12336=CARTESIAN_POINT('',(15.49,4.,2.89));
#12337=CARTESIAN_POINT('Origin',(15.5,4.15,2.98));
#12338=CARTESIAN_POINT('',(8.25,4.,2.98));
#12339=CARTESIAN_POINT('Origin',(14.51,4.3,2.98));
#12340=CARTESIAN_POINT('',(14.51,4.3,2.98));
#12341=CARTESIAN_POINT('',(14.49,4.3,2.98));
#12342=CARTESIAN_POINT('',(14.51,4.3,2.98));
#12343=CARTESIAN_POINT('',(14.51,4.3,3.));
#12344=CARTESIAN_POINT('',(14.51,4.3,2.98));
#12345=CARTESIAN_POINT('',(14.49,4.3,3.));
#12346=CARTESIAN_POINT('',(12.755,4.3,3.));
#12347=CARTESIAN_POINT('',(14.49,4.3,2.98));
#12348=CARTESIAN_POINT('Origin',(14.51,4.,2.98));
#12349=CARTESIAN_POINT('',(14.51,4.,2.98));
#12350=CARTESIAN_POINT('',(14.51,4.,2.98));
#12351=CARTESIAN_POINT('',(14.51,4.,3.));
#12352=CARTESIAN_POINT('',(14.51,4.,2.89));
#12353=CARTESIAN_POINT('',(14.51,4.2,3.));
#12354=CARTESIAN_POINT('Origin',(14.49,4.3,2.98));
#12355=CARTESIAN_POINT('',(14.49,4.,2.98));
#12356=CARTESIAN_POINT('',(14.49,4.3,2.98));
#12357=CARTESIAN_POINT('',(14.49,4.,3.));
#12358=CARTESIAN_POINT('',(14.49,4.35,3.));
#12359=CARTESIAN_POINT('',(14.49,4.,2.89));
#12360=CARTESIAN_POINT('Origin',(14.5,4.15,2.98));
#12361=CARTESIAN_POINT('',(7.75,4.,2.98));
#12362=CARTESIAN_POINT('Origin',(13.51,4.3,2.98));
#12363=CARTESIAN_POINT('',(13.51,4.3,2.98));
#12364=CARTESIAN_POINT('',(13.49,4.3,2.98));
#12365=CARTESIAN_POINT('',(13.51,4.3,2.98));
#12366=CARTESIAN_POINT('',(13.51,4.3,3.));
#12367=CARTESIAN_POINT('',(13.51,4.3,2.98));
#12368=CARTESIAN_POINT('',(13.49,4.3,3.));
#12369=CARTESIAN_POINT('',(12.255,4.3,3.));
#12370=CARTESIAN_POINT('',(13.49,4.3,2.98));
#12371=CARTESIAN_POINT('Origin',(13.51,4.,2.98));
#12372=CARTESIAN_POINT('',(13.51,4.,2.98));
#12373=CARTESIAN_POINT('',(13.51,4.,2.98));
#12374=CARTESIAN_POINT('',(13.51,4.,3.));
#12375=CARTESIAN_POINT('',(13.51,4.,2.89));
#12376=CARTESIAN_POINT('',(13.51,4.2,3.));
#12377=CARTESIAN_POINT('Origin',(13.49,4.3,2.98));
#12378=CARTESIAN_POINT('',(13.49,4.,2.98));
#12379=CARTESIAN_POINT('',(13.49,4.3,2.98));
#12380=CARTESIAN_POINT('',(13.49,4.,3.));
#12381=CARTESIAN_POINT('',(13.49,4.35,3.));
#12382=CARTESIAN_POINT('',(13.49,4.,2.89));
#12383=CARTESIAN_POINT('Origin',(13.5,4.15,2.98));
#12384=CARTESIAN_POINT('',(7.25,4.,2.98));
#12385=CARTESIAN_POINT('Origin',(12.51,4.3,2.98));
#12386=CARTESIAN_POINT('',(12.51,4.3,2.98));
#12387=CARTESIAN_POINT('',(12.49,4.3,2.98));
#12388=CARTESIAN_POINT('',(12.51,4.3,2.98));
#12389=CARTESIAN_POINT('',(12.51,4.3,3.));
#12390=CARTESIAN_POINT('',(12.51,4.3,2.98));
#12391=CARTESIAN_POINT('',(12.49,4.3,3.));
#12392=CARTESIAN_POINT('',(11.755,4.3,3.));
#12393=CARTESIAN_POINT('',(12.49,4.3,2.98));
#12394=CARTESIAN_POINT('Origin',(12.51,4.,2.98));
#12395=CARTESIAN_POINT('',(12.51,4.,2.98));
#12396=CARTESIAN_POINT('',(12.51,4.,2.98));
#12397=CARTESIAN_POINT('',(12.51,4.,3.));
#12398=CARTESIAN_POINT('',(12.51,4.,2.89));
#12399=CARTESIAN_POINT('',(12.51,4.2,3.));
#12400=CARTESIAN_POINT('Origin',(12.49,4.3,2.98));
#12401=CARTESIAN_POINT('',(12.49,4.,2.98));
#12402=CARTESIAN_POINT('',(12.49,4.3,2.98));
#12403=CARTESIAN_POINT('',(12.49,4.,3.));
#12404=CARTESIAN_POINT('',(12.49,4.35,3.));
#12405=CARTESIAN_POINT('',(12.49,4.,2.89));
#12406=CARTESIAN_POINT('Origin',(12.5,4.15,2.98));
#12407=CARTESIAN_POINT('',(6.75,4.,2.98));
#12408=CARTESIAN_POINT('Origin',(11.51,4.3,2.98));
#12409=CARTESIAN_POINT('',(11.51,4.3,2.98));
#12410=CARTESIAN_POINT('',(11.49,4.3,2.98));
#12411=CARTESIAN_POINT('',(11.51,4.3,2.98));
#12412=CARTESIAN_POINT('',(11.51,4.3,3.));
#12413=CARTESIAN_POINT('',(11.51,4.3,2.98));
#12414=CARTESIAN_POINT('',(11.49,4.3,3.));
#12415=CARTESIAN_POINT('',(11.255,4.3,3.));
#12416=CARTESIAN_POINT('',(11.49,4.3,2.98));
#12417=CARTESIAN_POINT('Origin',(11.51,4.,2.98));
#12418=CARTESIAN_POINT('',(11.51,4.,2.98));
#12419=CARTESIAN_POINT('',(11.51,4.,2.98));
#12420=CARTESIAN_POINT('',(11.51,4.,3.));
#12421=CARTESIAN_POINT('',(11.51,4.,2.89));
#12422=CARTESIAN_POINT('',(11.51,4.2,3.));
#12423=CARTESIAN_POINT('Origin',(11.49,4.3,2.98));
#12424=CARTESIAN_POINT('',(11.49,4.,2.98));
#12425=CARTESIAN_POINT('',(11.49,4.3,2.98));
#12426=CARTESIAN_POINT('',(11.49,4.,3.));
#12427=CARTESIAN_POINT('',(11.49,4.35,3.));
#12428=CARTESIAN_POINT('',(11.49,4.,2.89));
#12429=CARTESIAN_POINT('Origin',(11.5,4.15,2.98));
#12430=CARTESIAN_POINT('',(6.25,4.,2.98));
#12431=CARTESIAN_POINT('Origin',(11.01,4.5,2.98));
#12432=CARTESIAN_POINT('',(11.01,4.5,2.98));
#12433=CARTESIAN_POINT('',(10.99,4.5,2.98));
#12434=CARTESIAN_POINT('',(11.01,4.5,2.98));
#12435=CARTESIAN_POINT('',(11.01,4.5,3.));
#12436=CARTESIAN_POINT('',(11.01,4.5,2.98));
#12437=CARTESIAN_POINT('',(10.99,4.5,3.));
#12438=CARTESIAN_POINT('',(11.005,4.5,3.));
#12439=CARTESIAN_POINT('',(10.99,4.5,2.98));
#12440=CARTESIAN_POINT('Origin',(11.01,4.,2.98));
#12441=CARTESIAN_POINT('',(11.01,4.,2.98));
#12442=CARTESIAN_POINT('',(11.01,4.,2.98));
#12443=CARTESIAN_POINT('',(11.01,4.,3.));
#12444=CARTESIAN_POINT('',(11.01,4.,2.89));
#12445=CARTESIAN_POINT('',(11.01,4.2,3.));
#12446=CARTESIAN_POINT('Origin',(10.99,4.5,2.98));
#12447=CARTESIAN_POINT('',(10.99,4.,2.98));
#12448=CARTESIAN_POINT('',(10.99,4.5,2.98));
#12449=CARTESIAN_POINT('',(10.99,4.,3.));
#12450=CARTESIAN_POINT('',(10.99,4.45,3.));
#12451=CARTESIAN_POINT('',(10.99,4.,2.89));
#12452=CARTESIAN_POINT('Origin',(11.,4.25,2.98));
#12453=CARTESIAN_POINT('',(6.,4.,2.98));
#12454=CARTESIAN_POINT('Origin',(10.01,4.5,2.98));
#12455=CARTESIAN_POINT('',(10.01,4.5,2.98));
#12456=CARTESIAN_POINT('',(9.99,4.5,2.98));
#12457=CARTESIAN_POINT('',(10.01,4.5,2.98));
#12458=CARTESIAN_POINT('',(10.01,4.5,3.));
#12459=CARTESIAN_POINT('',(10.01,4.5,2.98));
#12460=CARTESIAN_POINT('',(9.99,4.5,3.));
#12461=CARTESIAN_POINT('',(10.505,4.5,3.));
#12462=CARTESIAN_POINT('',(9.99,4.5,2.98));
#12463=CARTESIAN_POINT('Origin',(10.01,4.,2.98));
#12464=CARTESIAN_POINT('',(10.01,4.,2.98));
#12465=CARTESIAN_POINT('',(10.01,4.,2.98));
#12466=CARTESIAN_POINT('',(10.01,4.,3.));
#12467=CARTESIAN_POINT('',(10.01,4.,2.89));
#12468=CARTESIAN_POINT('',(10.01,4.2,3.));
#12469=CARTESIAN_POINT('Origin',(9.99,4.5,2.98));
#12470=CARTESIAN_POINT('',(9.99,4.,2.98));
#12471=CARTESIAN_POINT('',(9.99,4.5,2.98));
#12472=CARTESIAN_POINT('',(9.99,4.,3.));
#12473=CARTESIAN_POINT('',(9.99,4.45,3.));
#12474=CARTESIAN_POINT('',(9.99,4.,2.89));
#12475=CARTESIAN_POINT('Origin',(10.,4.25,2.98));
#12476=CARTESIAN_POINT('',(5.5,4.,2.98));
#12477=CARTESIAN_POINT('Origin',(9.01,4.5,2.98));
#12478=CARTESIAN_POINT('',(9.01,4.5,2.98));
#12479=CARTESIAN_POINT('',(8.99,4.5,2.98));
#12480=CARTESIAN_POINT('',(9.01,4.5,2.98));
#12481=CARTESIAN_POINT('',(9.01,4.5,3.));
#12482=CARTESIAN_POINT('',(9.01,4.5,2.98));
#12483=CARTESIAN_POINT('',(8.99,4.5,3.));
#12484=CARTESIAN_POINT('',(10.005,4.5,3.));
#12485=CARTESIAN_POINT('',(8.99,4.5,2.98));
#12486=CARTESIAN_POINT('Origin',(9.01,4.,2.98));
#12487=CARTESIAN_POINT('',(9.01,4.,2.98));
#12488=CARTESIAN_POINT('',(9.01,4.,2.98));
#12489=CARTESIAN_POINT('',(9.01,4.,3.));
#12490=CARTESIAN_POINT('',(9.01,4.,2.89));
#12491=CARTESIAN_POINT('',(9.01,4.2,3.));
#12492=CARTESIAN_POINT('Origin',(8.99,4.5,2.98));
#12493=CARTESIAN_POINT('',(8.99,4.,2.98));
#12494=CARTESIAN_POINT('',(8.99,4.5,2.98));
#12495=CARTESIAN_POINT('',(8.99,4.,3.));
#12496=CARTESIAN_POINT('',(8.99,4.45,3.));
#12497=CARTESIAN_POINT('',(8.99,4.,2.89));
#12498=CARTESIAN_POINT('Origin',(9.,4.25,2.98));
#12499=CARTESIAN_POINT('',(5.,4.,2.98));
#12500=CARTESIAN_POINT('Origin',(8.01,4.5,2.98));
#12501=CARTESIAN_POINT('',(8.01,4.5,2.98));
#12502=CARTESIAN_POINT('',(7.99,4.5,2.98));
#12503=CARTESIAN_POINT('',(8.01,4.5,2.98));
#12504=CARTESIAN_POINT('',(8.01,4.5,3.));
#12505=CARTESIAN_POINT('',(8.01,4.5,2.98));
#12506=CARTESIAN_POINT('',(7.99,4.5,3.));
#12507=CARTESIAN_POINT('',(9.505,4.5,3.));
#12508=CARTESIAN_POINT('',(7.99,4.5,2.98));
#12509=CARTESIAN_POINT('Origin',(8.01,4.,2.98));
#12510=CARTESIAN_POINT('',(8.01,4.,2.98));
#12511=CARTESIAN_POINT('',(8.01,4.,2.98));
#12512=CARTESIAN_POINT('',(8.01,4.,3.));
#12513=CARTESIAN_POINT('',(8.01,4.,2.89));
#12514=CARTESIAN_POINT('',(8.01,4.2,3.));
#12515=CARTESIAN_POINT('Origin',(7.99,4.5,2.98));
#12516=CARTESIAN_POINT('',(7.99,4.,2.98));
#12517=CARTESIAN_POINT('',(7.99,4.5,2.98));
#12518=CARTESIAN_POINT('',(7.99,4.,3.));
#12519=CARTESIAN_POINT('',(7.99,4.45,3.));
#12520=CARTESIAN_POINT('',(7.99,4.,2.89));
#12521=CARTESIAN_POINT('Origin',(8.,4.25,2.98));
#12522=CARTESIAN_POINT('',(4.5,4.,2.98));
#12523=CARTESIAN_POINT('Origin',(7.01,4.5,2.98));
#12524=CARTESIAN_POINT('',(7.01,4.5,2.98));
#12525=CARTESIAN_POINT('',(6.99,4.5,2.98));
#12526=CARTESIAN_POINT('',(7.01,4.5,2.98));
#12527=CARTESIAN_POINT('',(7.01,4.5,3.));
#12528=CARTESIAN_POINT('',(7.01,4.5,2.98));
#12529=CARTESIAN_POINT('',(6.99,4.5,3.));
#12530=CARTESIAN_POINT('',(9.005,4.5,3.));
#12531=CARTESIAN_POINT('',(6.99,4.5,2.98));
#12532=CARTESIAN_POINT('Origin',(7.01,4.,2.98));
#12533=CARTESIAN_POINT('',(7.01,4.,2.98));
#12534=CARTESIAN_POINT('',(7.01,4.,2.98));
#12535=CARTESIAN_POINT('',(7.01,4.,3.));
#12536=CARTESIAN_POINT('',(7.01,4.,2.89));
#12537=CARTESIAN_POINT('',(7.01,4.2,3.));
#12538=CARTESIAN_POINT('Origin',(6.99,4.5,2.98));
#12539=CARTESIAN_POINT('',(6.99,4.,2.98));
#12540=CARTESIAN_POINT('',(6.99,4.5,2.98));
#12541=CARTESIAN_POINT('',(6.99,4.,3.));
#12542=CARTESIAN_POINT('',(6.99,4.45,3.));
#12543=CARTESIAN_POINT('',(6.99,4.,2.89));
#12544=CARTESIAN_POINT('Origin',(7.,4.25,2.98));
#12545=CARTESIAN_POINT('',(4.,4.,2.98));
#12546=CARTESIAN_POINT('Origin',(6.01,4.5,2.98));
#12547=CARTESIAN_POINT('',(6.01,4.5,2.98));
#12548=CARTESIAN_POINT('',(5.99,4.5,2.98));
#12549=CARTESIAN_POINT('',(6.01,4.5,2.98));
#12550=CARTESIAN_POINT('',(6.01,4.5,3.));
#12551=CARTESIAN_POINT('',(6.01,4.5,2.98));
#12552=CARTESIAN_POINT('',(5.99,4.5,3.));
#12553=CARTESIAN_POINT('',(8.505,4.5,3.));
#12554=CARTESIAN_POINT('',(5.99,4.5,2.98));
#12555=CARTESIAN_POINT('Origin',(6.01,4.,2.98));
#12556=CARTESIAN_POINT('',(6.01,4.,2.98));
#12557=CARTESIAN_POINT('',(6.01,4.,2.98));
#12558=CARTESIAN_POINT('',(6.01,4.,3.));
#12559=CARTESIAN_POINT('',(6.01,4.,2.89));
#12560=CARTESIAN_POINT('',(6.01,4.2,3.));
#12561=CARTESIAN_POINT('Origin',(5.99,4.5,2.98));
#12562=CARTESIAN_POINT('',(5.99,4.,2.98));
#12563=CARTESIAN_POINT('',(5.99,4.5,2.98));
#12564=CARTESIAN_POINT('',(5.99,4.,3.));
#12565=CARTESIAN_POINT('',(5.99,4.45,3.));
#12566=CARTESIAN_POINT('',(5.99,4.,2.89));
#12567=CARTESIAN_POINT('Origin',(6.,4.25,2.98));
#12568=CARTESIAN_POINT('',(3.5,4.,2.98));
#12569=CARTESIAN_POINT('Origin',(5.01,4.5,2.98));
#12570=CARTESIAN_POINT('',(5.01,4.5,2.98));
#12571=CARTESIAN_POINT('',(4.99,4.5,2.98));
#12572=CARTESIAN_POINT('',(5.01,4.5,2.98));
#12573=CARTESIAN_POINT('',(5.01,4.5,3.));
#12574=CARTESIAN_POINT('',(5.01,4.5,2.98));
#12575=CARTESIAN_POINT('',(4.99,4.5,3.));
#12576=CARTESIAN_POINT('',(8.005,4.5,3.));
#12577=CARTESIAN_POINT('',(4.99,4.5,2.98));
#12578=CARTESIAN_POINT('Origin',(5.01,4.,2.98));
#12579=CARTESIAN_POINT('',(5.01,4.,2.98));
#12580=CARTESIAN_POINT('',(5.01,4.,2.98));
#12581=CARTESIAN_POINT('',(5.01,4.,3.));
#12582=CARTESIAN_POINT('',(5.01,4.,2.89));
#12583=CARTESIAN_POINT('',(5.01,4.2,3.));
#12584=CARTESIAN_POINT('Origin',(4.99,4.5,2.98));
#12585=CARTESIAN_POINT('',(4.99,4.,2.98));
#12586=CARTESIAN_POINT('',(4.99,4.5,2.98));
#12587=CARTESIAN_POINT('',(4.99,4.,3.));
#12588=CARTESIAN_POINT('',(4.99,4.45,3.));
#12589=CARTESIAN_POINT('',(4.99,4.,2.89));
#12590=CARTESIAN_POINT('Origin',(5.,4.25,2.98));
#12591=CARTESIAN_POINT('',(3.,4.,2.98));
#12592=CARTESIAN_POINT('Origin',(4.51,4.3,2.98));
#12593=CARTESIAN_POINT('',(4.51,4.3,2.98));
#12594=CARTESIAN_POINT('',(4.49,4.3,2.98));
#12595=CARTESIAN_POINT('',(4.51,4.3,2.98));
#12596=CARTESIAN_POINT('',(4.51,4.3,3.));
#12597=CARTESIAN_POINT('',(4.51,4.3,2.98));
#12598=CARTESIAN_POINT('',(4.49,4.3,3.));
#12599=CARTESIAN_POINT('',(7.755,4.3,3.));
#12600=CARTESIAN_POINT('',(4.49,4.3,2.98));
#12601=CARTESIAN_POINT('Origin',(4.51,4.,2.98));
#12602=CARTESIAN_POINT('',(4.51,4.,2.98));
#12603=CARTESIAN_POINT('',(4.51,4.,2.98));
#12604=CARTESIAN_POINT('',(4.51,4.,3.));
#12605=CARTESIAN_POINT('',(4.51,4.,2.89));
#12606=CARTESIAN_POINT('',(4.51,4.2,3.));
#12607=CARTESIAN_POINT('Origin',(4.49,4.3,2.98));
#12608=CARTESIAN_POINT('',(4.49,4.,2.98));
#12609=CARTESIAN_POINT('',(4.49,4.3,2.98));
#12610=CARTESIAN_POINT('',(4.49,4.,3.));
#12611=CARTESIAN_POINT('',(4.49,4.35,3.));
#12612=CARTESIAN_POINT('',(4.49,4.,2.89));
#12613=CARTESIAN_POINT('Origin',(4.5,4.15,2.98));
#12614=CARTESIAN_POINT('',(2.75,4.,2.98));
#12615=CARTESIAN_POINT('Origin',(5.51,4.3,2.98));
#12616=CARTESIAN_POINT('',(5.51,4.3,2.98));
#12617=CARTESIAN_POINT('',(5.49,4.3,2.98));
#12618=CARTESIAN_POINT('',(5.51,4.3,2.98));
#12619=CARTESIAN_POINT('',(5.51,4.3,3.));
#12620=CARTESIAN_POINT('',(5.51,4.3,2.98));
#12621=CARTESIAN_POINT('',(5.49,4.3,3.));
#12622=CARTESIAN_POINT('',(8.255,4.3,3.));
#12623=CARTESIAN_POINT('',(5.49,4.3,2.98));
#12624=CARTESIAN_POINT('Origin',(5.51,4.,2.98));
#12625=CARTESIAN_POINT('',(5.51,4.,2.98));
#12626=CARTESIAN_POINT('',(5.51,4.,2.98));
#12627=CARTESIAN_POINT('',(5.51,4.,3.));
#12628=CARTESIAN_POINT('',(5.51,4.,2.89));
#12629=CARTESIAN_POINT('',(5.51,4.2,3.));
#12630=CARTESIAN_POINT('Origin',(5.49,4.3,2.98));
#12631=CARTESIAN_POINT('',(5.49,4.,2.98));
#12632=CARTESIAN_POINT('',(5.49,4.3,2.98));
#12633=CARTESIAN_POINT('',(5.49,4.,3.));
#12634=CARTESIAN_POINT('',(5.49,4.35,3.));
#12635=CARTESIAN_POINT('',(5.49,4.,2.89));
#12636=CARTESIAN_POINT('Origin',(5.5,4.15,2.98));
#12637=CARTESIAN_POINT('',(3.25,4.,2.98));
#12638=CARTESIAN_POINT('Origin',(6.51,4.3,2.98));
#12639=CARTESIAN_POINT('',(6.51,4.3,2.98));
#12640=CARTESIAN_POINT('',(6.49,4.3,2.98));
#12641=CARTESIAN_POINT('',(6.51,4.3,2.98));
#12642=CARTESIAN_POINT('',(6.51,4.3,3.));
#12643=CARTESIAN_POINT('',(6.51,4.3,2.98));
#12644=CARTESIAN_POINT('',(6.49,4.3,3.));
#12645=CARTESIAN_POINT('',(8.755,4.3,3.));
#12646=CARTESIAN_POINT('',(6.49,4.3,2.98));
#12647=CARTESIAN_POINT('Origin',(6.51,4.,2.98));
#12648=CARTESIAN_POINT('',(6.51,4.,2.98));
#12649=CARTESIAN_POINT('',(6.51,4.,2.98));
#12650=CARTESIAN_POINT('',(6.51,4.,3.));
#12651=CARTESIAN_POINT('',(6.51,4.,2.89));
#12652=CARTESIAN_POINT('',(6.51,4.2,3.));
#12653=CARTESIAN_POINT('Origin',(6.49,4.3,2.98));
#12654=CARTESIAN_POINT('',(6.49,4.,2.98));
#12655=CARTESIAN_POINT('',(6.49,4.3,2.98));
#12656=CARTESIAN_POINT('',(6.49,4.,3.));
#12657=CARTESIAN_POINT('',(6.49,4.35,3.));
#12658=CARTESIAN_POINT('',(6.49,4.,2.89));
#12659=CARTESIAN_POINT('Origin',(6.5,4.15,2.98));
#12660=CARTESIAN_POINT('',(3.75,4.,2.98));
#12661=CARTESIAN_POINT('Origin',(7.51,4.3,2.98));
#12662=CARTESIAN_POINT('',(7.51,4.3,2.98));
#12663=CARTESIAN_POINT('',(7.49,4.3,2.98));
#12664=CARTESIAN_POINT('',(7.51,4.3,2.98));
#12665=CARTESIAN_POINT('',(7.51,4.3,3.));
#12666=CARTESIAN_POINT('',(7.51,4.3,2.98));
#12667=CARTESIAN_POINT('',(7.49,4.3,3.));
#12668=CARTESIAN_POINT('',(9.255,4.3,3.));
#12669=CARTESIAN_POINT('',(7.49,4.3,2.98));
#12670=CARTESIAN_POINT('Origin',(7.51,4.,2.98));
#12671=CARTESIAN_POINT('',(7.51,4.,2.98));
#12672=CARTESIAN_POINT('',(7.51,4.,2.98));
#12673=CARTESIAN_POINT('',(7.51,4.,3.));
#12674=CARTESIAN_POINT('',(7.51,4.,2.89));
#12675=CARTESIAN_POINT('',(7.51,4.2,3.));
#12676=CARTESIAN_POINT('Origin',(7.49,4.3,2.98));
#12677=CARTESIAN_POINT('',(7.49,4.,2.98));
#12678=CARTESIAN_POINT('',(7.49,4.3,2.98));
#12679=CARTESIAN_POINT('',(7.49,4.,3.));
#12680=CARTESIAN_POINT('',(7.49,4.35,3.));
#12681=CARTESIAN_POINT('',(7.49,4.,2.89));
#12682=CARTESIAN_POINT('Origin',(7.5,4.15,2.98));
#12683=CARTESIAN_POINT('',(4.25,4.,2.98));
#12684=CARTESIAN_POINT('Origin',(8.51,4.3,2.98));
#12685=CARTESIAN_POINT('',(8.51,4.3,2.98));
#12686=CARTESIAN_POINT('',(8.49,4.3,2.98));
#12687=CARTESIAN_POINT('',(8.51,4.3,2.98));
#12688=CARTESIAN_POINT('',(8.51,4.3,3.));
#12689=CARTESIAN_POINT('',(8.51,4.3,2.98));
#12690=CARTESIAN_POINT('',(8.49,4.3,3.));
#12691=CARTESIAN_POINT('',(9.755,4.3,3.));
#12692=CARTESIAN_POINT('',(8.49,4.3,2.98));
#12693=CARTESIAN_POINT('Origin',(8.51,4.,2.98));
#12694=CARTESIAN_POINT('',(8.51,4.,2.98));
#12695=CARTESIAN_POINT('',(8.51,4.,2.98));
#12696=CARTESIAN_POINT('',(8.51,4.,3.));
#12697=CARTESIAN_POINT('',(8.51,4.,2.89));
#12698=CARTESIAN_POINT('',(8.51,4.2,3.));
#12699=CARTESIAN_POINT('Origin',(8.49,4.3,2.98));
#12700=CARTESIAN_POINT('',(8.49,4.,2.98));
#12701=CARTESIAN_POINT('',(8.49,4.3,2.98));
#12702=CARTESIAN_POINT('',(8.49,4.,3.));
#12703=CARTESIAN_POINT('',(8.49,4.35,3.));
#12704=CARTESIAN_POINT('',(8.49,4.,2.89));
#12705=CARTESIAN_POINT('Origin',(8.5,4.15,2.98));
#12706=CARTESIAN_POINT('',(4.75,4.,2.98));
#12707=CARTESIAN_POINT('Origin',(9.51,4.3,2.98));
#12708=CARTESIAN_POINT('',(9.51,4.3,2.98));
#12709=CARTESIAN_POINT('',(9.49,4.3,2.98));
#12710=CARTESIAN_POINT('',(9.51,4.3,2.98));
#12711=CARTESIAN_POINT('',(9.51,4.3,3.));
#12712=CARTESIAN_POINT('',(9.51,4.3,2.98));
#12713=CARTESIAN_POINT('',(9.49,4.3,3.));
#12714=CARTESIAN_POINT('',(10.255,4.3,3.));
#12715=CARTESIAN_POINT('',(9.49,4.3,2.98));
#12716=CARTESIAN_POINT('Origin',(9.51,4.,2.98));
#12717=CARTESIAN_POINT('',(9.51,4.,2.98));
#12718=CARTESIAN_POINT('',(9.51,4.,2.98));
#12719=CARTESIAN_POINT('',(9.51,4.,3.));
#12720=CARTESIAN_POINT('',(9.51,4.,2.89));
#12721=CARTESIAN_POINT('',(9.51,4.2,3.));
#12722=CARTESIAN_POINT('Origin',(9.49,4.3,2.98));
#12723=CARTESIAN_POINT('',(9.49,4.,2.98));
#12724=CARTESIAN_POINT('',(9.49,4.3,2.98));
#12725=CARTESIAN_POINT('',(9.49,4.,3.));
#12726=CARTESIAN_POINT('',(9.49,4.35,3.));
#12727=CARTESIAN_POINT('',(9.49,4.,2.89));
#12728=CARTESIAN_POINT('Origin',(9.5,4.15,2.98));
#12729=CARTESIAN_POINT('',(5.25,4.,2.98));
#12730=CARTESIAN_POINT('Origin',(10.51,4.3,2.98));
#12731=CARTESIAN_POINT('',(10.51,4.3,2.98));
#12732=CARTESIAN_POINT('',(10.49,4.3,2.98));
#12733=CARTESIAN_POINT('',(10.51,4.3,2.98));
#12734=CARTESIAN_POINT('',(10.51,4.3,3.));
#12735=CARTESIAN_POINT('',(10.51,4.3,2.98));
#12736=CARTESIAN_POINT('',(10.49,4.3,3.));
#12737=CARTESIAN_POINT('',(10.755,4.3,3.));
#12738=CARTESIAN_POINT('',(10.49,4.3,2.98));
#12739=CARTESIAN_POINT('Origin',(10.51,4.,2.98));
#12740=CARTESIAN_POINT('',(10.51,4.,2.98));
#12741=CARTESIAN_POINT('',(10.51,4.,2.98));
#12742=CARTESIAN_POINT('',(10.51,4.,3.));
#12743=CARTESIAN_POINT('',(10.51,4.,2.89));
#12744=CARTESIAN_POINT('',(10.51,4.2,3.));
#12745=CARTESIAN_POINT('Origin',(10.49,4.3,2.98));
#12746=CARTESIAN_POINT('',(10.49,4.,2.98));
#12747=CARTESIAN_POINT('',(10.49,4.3,2.98));
#12748=CARTESIAN_POINT('',(10.49,4.,3.));
#12749=CARTESIAN_POINT('',(10.49,4.35,3.));
#12750=CARTESIAN_POINT('',(10.49,4.,2.89));
#12751=CARTESIAN_POINT('Origin',(10.5,4.15,2.98));
#12752=CARTESIAN_POINT('',(5.75,4.,2.98));
#12753=CARTESIAN_POINT('Origin',(4.01,4.5,2.98));
#12754=CARTESIAN_POINT('',(4.01,4.5,2.98));
#12755=CARTESIAN_POINT('',(3.99,4.5,2.98));
#12756=CARTESIAN_POINT('',(4.01,4.5,2.98));
#12757=CARTESIAN_POINT('',(4.01,4.5,3.));
#12758=CARTESIAN_POINT('',(4.01,4.5,2.98));
#12759=CARTESIAN_POINT('',(3.99,4.5,3.));
#12760=CARTESIAN_POINT('',(7.505,4.5,3.));
#12761=CARTESIAN_POINT('',(3.99,4.5,2.98));
#12762=CARTESIAN_POINT('Origin',(4.01,4.,2.98));
#12763=CARTESIAN_POINT('',(4.01,4.,2.98));
#12764=CARTESIAN_POINT('',(4.01,4.,2.98));
#12765=CARTESIAN_POINT('',(4.01,4.,3.));
#12766=CARTESIAN_POINT('',(4.01,4.,2.89));
#12767=CARTESIAN_POINT('',(4.01,4.2,3.));
#12768=CARTESIAN_POINT('Origin',(3.99,4.5,2.98));
#12769=CARTESIAN_POINT('',(3.99,4.,2.98));
#12770=CARTESIAN_POINT('',(3.99,4.5,2.98));
#12771=CARTESIAN_POINT('',(3.99,4.,3.));
#12772=CARTESIAN_POINT('',(3.99,4.45,3.));
#12773=CARTESIAN_POINT('',(3.99,4.,2.89));
#12774=CARTESIAN_POINT('Origin',(4.,4.25,2.98));
#12775=CARTESIAN_POINT('',(2.5,4.,2.98));
#12776=CARTESIAN_POINT('Origin',(12.01,4.5,2.98));
#12777=CARTESIAN_POINT('',(12.01,4.5,2.98));
#12778=CARTESIAN_POINT('',(11.99,4.5,2.98));
#12779=CARTESIAN_POINT('',(12.01,4.5,2.98));
#12780=CARTESIAN_POINT('',(12.01,4.5,3.));
#12781=CARTESIAN_POINT('',(12.01,4.5,2.98));
#12782=CARTESIAN_POINT('',(11.99,4.5,3.));
#12783=CARTESIAN_POINT('',(11.505,4.5,3.));
#12784=CARTESIAN_POINT('',(11.99,4.5,2.98));
#12785=CARTESIAN_POINT('Origin',(12.01,4.,2.98));
#12786=CARTESIAN_POINT('',(12.01,4.,2.98));
#12787=CARTESIAN_POINT('',(12.01,4.,2.98));
#12788=CARTESIAN_POINT('',(12.01,4.,3.));
#12789=CARTESIAN_POINT('',(12.01,4.,2.89));
#12790=CARTESIAN_POINT('',(12.01,4.2,3.));
#12791=CARTESIAN_POINT('Origin',(11.99,4.5,2.98));
#12792=CARTESIAN_POINT('',(11.99,4.,2.98));
#12793=CARTESIAN_POINT('',(11.99,4.5,2.98));
#12794=CARTESIAN_POINT('',(11.99,4.,3.));
#12795=CARTESIAN_POINT('',(11.99,4.45,3.));
#12796=CARTESIAN_POINT('',(11.99,4.,2.89));
#12797=CARTESIAN_POINT('Origin',(12.,4.25,2.98));
#12798=CARTESIAN_POINT('',(6.5,4.,2.98));
#12799=CARTESIAN_POINT('Origin',(13.01,4.5,2.98));
#12800=CARTESIAN_POINT('',(13.01,4.5,2.98));
#12801=CARTESIAN_POINT('',(12.99,4.5,2.98));
#12802=CARTESIAN_POINT('',(13.01,4.5,2.98));
#12803=CARTESIAN_POINT('',(13.01,4.5,3.));
#12804=CARTESIAN_POINT('',(13.01,4.5,2.98));
#12805=CARTESIAN_POINT('',(12.99,4.5,3.));
#12806=CARTESIAN_POINT('',(12.005,4.5,3.));
#12807=CARTESIAN_POINT('',(12.99,4.5,2.98));
#12808=CARTESIAN_POINT('Origin',(13.01,4.,2.98));
#12809=CARTESIAN_POINT('',(13.01,4.,2.98));
#12810=CARTESIAN_POINT('',(13.01,4.,2.98));
#12811=CARTESIAN_POINT('',(13.01,4.,3.));
#12812=CARTESIAN_POINT('',(13.01,4.,2.89));
#12813=CARTESIAN_POINT('',(13.01,4.2,3.));
#12814=CARTESIAN_POINT('Origin',(12.99,4.5,2.98));
#12815=CARTESIAN_POINT('',(12.99,4.,2.98));
#12816=CARTESIAN_POINT('',(12.99,4.5,2.98));
#12817=CARTESIAN_POINT('',(12.99,4.,3.));
#12818=CARTESIAN_POINT('',(12.99,4.45,3.));
#12819=CARTESIAN_POINT('',(12.99,4.,2.89));
#12820=CARTESIAN_POINT('Origin',(13.,4.25,2.98));
#12821=CARTESIAN_POINT('',(7.,4.,2.98));
#12822=CARTESIAN_POINT('Origin',(14.01,4.5,2.98));
#12823=CARTESIAN_POINT('',(14.01,4.5,2.98));
#12824=CARTESIAN_POINT('',(13.99,4.5,2.98));
#12825=CARTESIAN_POINT('',(14.01,4.5,2.98));
#12826=CARTESIAN_POINT('',(14.01,4.5,3.));
#12827=CARTESIAN_POINT('',(14.01,4.5,2.98));
#12828=CARTESIAN_POINT('',(13.99,4.5,3.));
#12829=CARTESIAN_POINT('',(12.505,4.5,3.));
#12830=CARTESIAN_POINT('',(13.99,4.5,2.98));
#12831=CARTESIAN_POINT('Origin',(14.01,4.,2.98));
#12832=CARTESIAN_POINT('',(14.01,4.,2.98));
#12833=CARTESIAN_POINT('',(14.01,4.,2.98));
#12834=CARTESIAN_POINT('',(14.01,4.,3.));
#12835=CARTESIAN_POINT('',(14.01,4.,2.89));
#12836=CARTESIAN_POINT('',(14.01,4.2,3.));
#12837=CARTESIAN_POINT('Origin',(13.99,4.5,2.98));
#12838=CARTESIAN_POINT('',(13.99,4.,2.98));
#12839=CARTESIAN_POINT('',(13.99,4.5,2.98));
#12840=CARTESIAN_POINT('',(13.99,4.,3.));
#12841=CARTESIAN_POINT('',(13.99,4.45,3.));
#12842=CARTESIAN_POINT('',(13.99,4.,2.89));
#12843=CARTESIAN_POINT('Origin',(14.,4.25,2.98));
#12844=CARTESIAN_POINT('',(7.5,4.,2.98));
#12845=CARTESIAN_POINT('Origin',(15.01,4.5,2.98));
#12846=CARTESIAN_POINT('',(15.01,4.5,2.98));
#12847=CARTESIAN_POINT('',(14.99,4.5,2.98));
#12848=CARTESIAN_POINT('',(15.01,4.5,2.98));
#12849=CARTESIAN_POINT('',(15.01,4.5,3.));
#12850=CARTESIAN_POINT('',(15.01,4.5,2.98));
#12851=CARTESIAN_POINT('',(14.99,4.5,3.));
#12852=CARTESIAN_POINT('',(13.005,4.5,3.));
#12853=CARTESIAN_POINT('',(14.99,4.5,2.98));
#12854=CARTESIAN_POINT('Origin',(15.01,4.,2.98));
#12855=CARTESIAN_POINT('',(15.01,4.,2.98));
#12856=CARTESIAN_POINT('',(15.01,4.,2.98));
#12857=CARTESIAN_POINT('',(15.01,4.,3.));
#12858=CARTESIAN_POINT('',(15.01,4.,2.89));
#12859=CARTESIAN_POINT('',(15.01,4.2,3.));
#12860=CARTESIAN_POINT('Origin',(14.99,4.5,2.98));
#12861=CARTESIAN_POINT('',(14.99,4.,2.98));
#12862=CARTESIAN_POINT('',(14.99,4.5,2.98));
#12863=CARTESIAN_POINT('',(14.99,4.,3.));
#12864=CARTESIAN_POINT('',(14.99,4.45,3.));
#12865=CARTESIAN_POINT('',(14.99,4.,2.89));
#12866=CARTESIAN_POINT('Origin',(15.,4.25,2.98));
#12867=CARTESIAN_POINT('',(8.,4.,2.98));
#12868=CARTESIAN_POINT('Origin',(16.01,4.5,2.98));
#12869=CARTESIAN_POINT('',(16.01,4.5,2.98));
#12870=CARTESIAN_POINT('',(15.99,4.5,2.98));
#12871=CARTESIAN_POINT('',(16.01,4.5,2.98));
#12872=CARTESIAN_POINT('',(16.01,4.5,3.));
#12873=CARTESIAN_POINT('',(16.01,4.5,2.98));
#12874=CARTESIAN_POINT('',(15.99,4.5,3.));
#12875=CARTESIAN_POINT('',(13.505,4.5,3.));
#12876=CARTESIAN_POINT('',(15.99,4.5,2.98));
#12877=CARTESIAN_POINT('Origin',(16.01,4.,2.98));
#12878=CARTESIAN_POINT('',(16.01,4.,2.98));
#12879=CARTESIAN_POINT('',(16.01,4.,2.98));
#12880=CARTESIAN_POINT('',(16.01,4.,3.));
#12881=CARTESIAN_POINT('',(16.01,4.,2.89));
#12882=CARTESIAN_POINT('',(16.01,4.2,3.));
#12883=CARTESIAN_POINT('Origin',(15.99,4.5,2.98));
#12884=CARTESIAN_POINT('',(15.99,4.,2.98));
#12885=CARTESIAN_POINT('',(15.99,4.5,2.98));
#12886=CARTESIAN_POINT('',(15.99,4.,3.));
#12887=CARTESIAN_POINT('',(15.99,4.45,3.));
#12888=CARTESIAN_POINT('',(15.99,4.,2.89));
#12889=CARTESIAN_POINT('Origin',(16.,4.25,2.98));
#12890=CARTESIAN_POINT('',(8.5,4.,2.98));
#12891=CARTESIAN_POINT('Origin',(17.01,4.5,2.98));
#12892=CARTESIAN_POINT('',(17.01,4.5,2.98));
#12893=CARTESIAN_POINT('',(16.99,4.5,2.98));
#12894=CARTESIAN_POINT('',(17.01,4.5,2.98));
#12895=CARTESIAN_POINT('',(17.01,4.5,3.));
#12896=CARTESIAN_POINT('',(17.01,4.5,2.98));
#12897=CARTESIAN_POINT('',(16.99,4.5,3.));
#12898=CARTESIAN_POINT('',(14.005,4.5,3.));
#12899=CARTESIAN_POINT('',(16.99,4.5,2.98));
#12900=CARTESIAN_POINT('Origin',(17.01,4.,2.98));
#12901=CARTESIAN_POINT('',(17.01,4.,2.98));
#12902=CARTESIAN_POINT('',(17.01,4.,2.98));
#12903=CARTESIAN_POINT('',(17.01,4.,3.));
#12904=CARTESIAN_POINT('',(17.01,4.,2.89));
#12905=CARTESIAN_POINT('',(17.01,4.2,3.));
#12906=CARTESIAN_POINT('Origin',(16.99,4.5,2.98));
#12907=CARTESIAN_POINT('',(16.99,4.,2.98));
#12908=CARTESIAN_POINT('',(16.99,4.5,2.98));
#12909=CARTESIAN_POINT('',(16.99,4.,3.));
#12910=CARTESIAN_POINT('',(16.99,4.45,3.));
#12911=CARTESIAN_POINT('',(16.99,4.,2.89));
#12912=CARTESIAN_POINT('Origin',(17.,4.25,2.98));
#12913=CARTESIAN_POINT('',(9.,4.,2.98));
#12914=CARTESIAN_POINT('Origin',(18.01,4.5,2.98));
#12915=CARTESIAN_POINT('',(18.01,4.5,2.98));
#12916=CARTESIAN_POINT('',(17.99,4.5,2.98));
#12917=CARTESIAN_POINT('',(18.01,4.5,2.98));
#12918=CARTESIAN_POINT('',(18.01,4.5,3.));
#12919=CARTESIAN_POINT('',(18.01,4.5,2.98));
#12920=CARTESIAN_POINT('',(17.99,4.5,3.));
#12921=CARTESIAN_POINT('',(14.505,4.5,3.));
#12922=CARTESIAN_POINT('',(17.99,4.5,2.98));
#12923=CARTESIAN_POINT('Origin',(18.01,4.,2.98));
#12924=CARTESIAN_POINT('',(18.01,4.,2.98));
#12925=CARTESIAN_POINT('',(18.01,4.,2.98));
#12926=CARTESIAN_POINT('',(18.01,4.,3.));
#12927=CARTESIAN_POINT('',(18.01,4.,2.89));
#12928=CARTESIAN_POINT('',(18.01,4.2,3.));
#12929=CARTESIAN_POINT('Origin',(17.99,4.5,2.98));
#12930=CARTESIAN_POINT('',(17.99,4.,2.98));
#12931=CARTESIAN_POINT('',(17.99,4.5,2.98));
#12932=CARTESIAN_POINT('',(17.99,4.,3.));
#12933=CARTESIAN_POINT('',(17.99,4.45,3.));
#12934=CARTESIAN_POINT('',(17.99,4.,2.89));
#12935=CARTESIAN_POINT('Origin',(18.,4.25,2.98));
#12936=CARTESIAN_POINT('',(9.5,4.,2.98));
#12937=CARTESIAN_POINT('Origin',(11.,4.4,3.));
#12938=CARTESIAN_POINT('',(1.,4.,3.));
#12939=CARTESIAN_POINT('',(21.,4.,3.));
#12940=CARTESIAN_POINT('',(1.,4.,3.));
#12941=CARTESIAN_POINT('',(21.,4.8,3.));
#12942=CARTESIAN_POINT('',(21.,4.,3.));
#12943=CARTESIAN_POINT('',(1.,4.8,3.));
#12944=CARTESIAN_POINT('',(21.,4.8,3.));
#12945=CARTESIAN_POINT('',(1.,4.,3.));
#12946=CARTESIAN_POINT('',(1.,4.8,3.));
#12947=CARTESIAN_POINT('',(1.,4.,3.));
#12948=CARTESIAN_POINT('',(1.,4.,3.));
#12949=CARTESIAN_POINT('',(1.,4.,3.));
#12950=CARTESIAN_POINT('',(1.,4.,3.));
#12951=CARTESIAN_POINT('',(1.,4.,3.));
#12952=CARTESIAN_POINT('',(1.,4.,3.));
#12953=CARTESIAN_POINT('',(1.,4.,3.));
#12954=CARTESIAN_POINT('',(1.,4.,3.));
#12955=CARTESIAN_POINT('',(1.,4.,3.));
#12956=CARTESIAN_POINT('',(1.,4.,3.));
#12957=CARTESIAN_POINT('',(1.,4.,3.));
#12958=CARTESIAN_POINT('',(1.,4.,3.));
#12959=CARTESIAN_POINT('',(1.,4.,3.));
#12960=CARTESIAN_POINT('',(1.,4.,3.));
#12961=CARTESIAN_POINT('',(1.,4.,3.));
#12962=CARTESIAN_POINT('',(1.,4.,3.));
#12963=CARTESIAN_POINT('',(1.,4.,3.));
#12964=CARTESIAN_POINT('',(1.,4.,3.));
#12965=CARTESIAN_POINT('',(1.,4.,3.));
#12966=CARTESIAN_POINT('',(1.,4.,3.));
#12967=CARTESIAN_POINT('',(1.,4.,3.));
#12968=CARTESIAN_POINT('',(1.,4.,3.));
#12969=CARTESIAN_POINT('',(1.,4.,3.));
#12970=CARTESIAN_POINT('',(1.,4.,3.));
#12971=CARTESIAN_POINT('',(1.,4.,3.));
#12972=CARTESIAN_POINT('',(1.,4.,3.));
#12973=CARTESIAN_POINT('',(1.,4.,3.));
#12974=CARTESIAN_POINT('',(1.,4.,3.));
#12975=CARTESIAN_POINT('',(19.775,4.4,3.));
#12976=CARTESIAN_POINT('Origin',(20.,4.4,3.));
#12977=CARTESIAN_POINT('',(1.775,4.4,3.));
#12978=CARTESIAN_POINT('Origin',(2.,4.4,3.));
#12979=CARTESIAN_POINT('Origin',(2.,4.4,2.7));
#12980=CARTESIAN_POINT('',(1.775,4.4,2.8));
#12981=CARTESIAN_POINT('Origin',(2.,4.4,2.8));
#12982=CARTESIAN_POINT('',(1.775,4.4,2.7));
#12983=CARTESIAN_POINT('Origin',(20.,4.4,2.7));
#12984=CARTESIAN_POINT('',(19.775,4.4,2.8));
#12985=CARTESIAN_POINT('Origin',(20.,4.4,2.8));
#12986=CARTESIAN_POINT('',(19.775,4.4,2.7));
#12987=CARTESIAN_POINT('Origin',(21.,4.8,2.8));
#12988=CARTESIAN_POINT('',(21.,4.8,2.8));
#12989=CARTESIAN_POINT('',(1.,4.8,2.8));
#12990=CARTESIAN_POINT('',(21.,4.8,2.8));
#12991=CARTESIAN_POINT('',(1.,4.8,2.8));
#12992=CARTESIAN_POINT('',(21.,4.8,2.8));
#12993=CARTESIAN_POINT('Origin',(21.,4.,2.8));
#12994=CARTESIAN_POINT('',(21.,4.,2.8));
#12995=CARTESIAN_POINT('',(21.,4.,2.8));
#12996=CARTESIAN_POINT('',(21.,4.,2.8));
#12997=CARTESIAN_POINT('Origin',(1.,4.,2.8));
#12998=CARTESIAN_POINT('',(1.,4.,2.8));
#12999=CARTESIAN_POINT('',(1.,4.,2.8));
#13000=CARTESIAN_POINT('',(1.,4.,2.8));
#13001=CARTESIAN_POINT('Origin',(1.,4.8,2.8));
#13002=CARTESIAN_POINT('',(1.,4.8,2.8));
#13003=CARTESIAN_POINT('Origin',(11.,4.4,2.8));
#14422=UNCERTAINTY_MEASURE_WITH_UNIT(LENGTH_MEASURE(0.001),#14479,
'DISTANCE_ACCURACY_VALUE',
'Maximum model space distance between geometric entities at asserted c
onnectivities');
#14446=UNCERTAINTY_MEASURE_WITH_UNIT(LENGTH_MEASURE(0.001),#14479,
'DISTANCE_ACCURACY_VALUE',
'Maximum model space distance between geometric entities at asserted c
onnectivities');
#14454=(
GEOMETRIC_REPRESENTATION_CONTEXT(3)
GLOBAL_UNCERTAINTY_ASSIGNED_CONTEXT((#14422))
GLOBAL_UNIT_ASSIGNED_CONTEXT((#14479,#14481,#14482))
REPRESENTATION_CONTEXT('','3D')
);
#14478=(
GEOMETRIC_REPRESENTATION_CONTEXT(3)
GLOBAL_UNCERTAINTY_ASSIGNED_CONTEXT((#14446))
GLOBAL_UNIT_ASSIGNED_CONTEXT((#14479,#14481,#14482))
REPRESENTATION_CONTEXT('','3D')
);
#14479=(
LENGTH_UNIT()
NAMED_UNIT(*)
SI_UNIT(.CENTI.,.METRE.)
);
#14481=(
NAMED_UNIT(*)
PLANE_ANGLE_UNIT()
SI_UNIT($,.RADIAN.)
);
#14482=(
NAMED_UNIT(*)
SI_UNIT($,.STERADIAN.)
SOLID_ANGLE_UNIT()
);
#14490=SHAPE_DEFINITION_REPRESENTATION(#14521,#14610);
#14521=PRODUCT_DEFINITION_SHAPE('',$,#14642);
#14610=SHAPE_REPRESENTATION('',(#9026),#14454);
#14634=PRODUCT_DEFINITION_CONTEXT('part definition',#14729,'design');
#14642=PRODUCT_DEFINITION('Graduated scale','Graduated scale',#14673,#14634);
#14673=PRODUCT_DEFINITION_FORMATION('',$,#14738);
#14729=APPLICATION_CONTEXT(
'Core Data for Automotive Mechanical Design Process');
#14730=PRODUCT_CONTEXT('part definition',#14729,'mechanical');
#14738=PRODUCT('Graduated scale','Graduated scale','Graduated scale',(#14730));
#14839=COLOUR_RGB('Off White',0.89,0.88,0.83);
#14840=FILL_AREA_STYLE_COLOUR('',#14839);
#14841=FILL_AREA_STYLE('',(#14840));
#14842=SURFACE_STYLE_FILL_AREA(#14841);
#14843=SURFACE_SIDE_STYLE('',(#14842));
#14844=SURFACE_STYLE_USAGE(.BOTH.,#14843);
#14845=PRESENTATION_STYLE_ASSIGNMENT((#14844));
ENDSEC;
END-ISO-10303-21;
